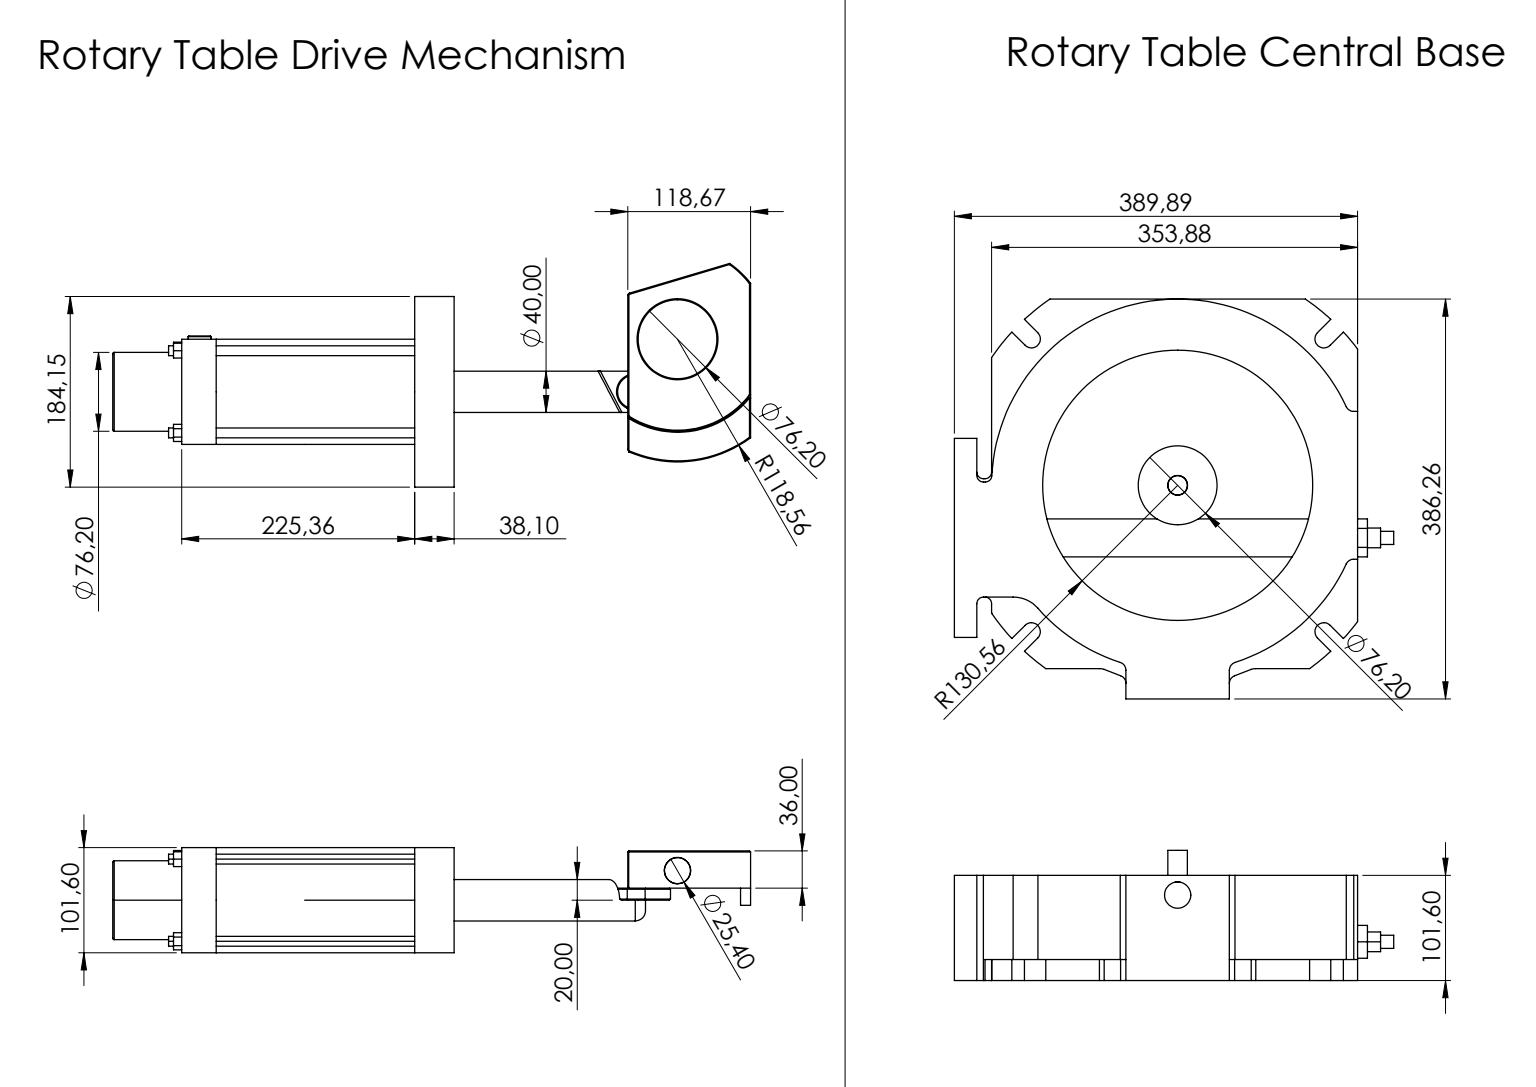
ISO-10303-21;
HEADER;
FILE_DESCRIPTION (('STEP AP214'),
    '1' );
FILE_NAME ('Rotary Table Drive Mechanism.step',
    '2026-10-07T11:37:37',
    ( '' ),
    ( '' ),
    'SwSTEP 2.0',
    'SolidWorks 2020',
    '' );
FILE_SCHEMA (( 'AUTOMOTIVE_DESIGN' ));
ENDSEC;

DATA;
#19=VERTEX_POINT ( 'NONE', #31186 ) ;
#30=CARTESIAN_POINT ( 'NONE',  ( 0.8292115003195463796, 69.84999999999999432, 118.5559999999999832 ) ) ;
#36=DIRECTION ( 'NONE',  ( 0.000000000000000000, 0.000000000000000000, -1.000000000000000000 ) ) ;
#65=DIRECTION ( 'NONE',  ( -0.7071067811865475727, -0.7071067811865475727, 0.000000000000000000 ) ) ;
#72=ADVANCED_FACE ( 'NONE', ( #9419 ), #85748, .F. ) ;
#76=AXIS2_PLACEMENT_3D ( 'NONE', #21854, #16377, #36372 ) ;
#122=DIRECTION ( 'NONE',  ( 0.000000000000000000, -1.000000000000000000, 0.000000000000000000 ) ) ;
#157=DIRECTION ( 'NONE',  ( 1.000000000000000000, 0.000000000000000000, 0.000000000000000000 ) ) ;
#176=DIRECTION ( 'NONE',  ( 1.000000000000000000, 0.000000000000000000, 1.821299053822143307E-16 ) ) ;
#194=AXIS2_PLACEMENT_3D ( 'NONE', #47993, #62984, #27575 ) ;
#207=DIRECTION ( 'NONE',  ( 1.000000000000000000, 0.000000000000000000, 0.000000000000000000 ) ) ;
#214=ORIENTED_EDGE ( 'NONE', *, *, #36681, .T. ) ;
#244=EDGE_CURVE ( 'NONE', #1586, #65784, #48833, .T. ) ;
#274=VERTEX_POINT ( 'NONE', #40238 ) ;
#280=EDGE_CURVE ( 'NONE', #76657, #85611, #63382, .T. ) ;
#296=VERTEX_POINT ( 'NONE', #28870 ) ;
#343=CARTESIAN_POINT ( 'NONE',  ( -479.3614999999999782, 100.8062500000000057, 94.61194598552329182 ) ) ;
#351=LINE ( 'NONE', #55290, #78955 ) ;
#356=DIRECTION ( 'NONE',  ( 0.000000000000000000, 0.000000000000000000, 1.000000000000000000 ) ) ;
#360=DIRECTION ( 'NONE',  ( 0.000000000000000000, 0.000000000000000000, -1.000000000000000000 ) ) ;
#382=EDGE_LOOP ( 'NONE', ( #48463, #62234, #46660, #29247, #79434, #62043 ) ) ;
#393=CARTESIAN_POINT ( 'NONE',  ( -487.2989999999999782, 14.28749999999982201, 90.48749999999999716 ) ) ;
#415=DIRECTION ( 'NONE',  ( 1.000000000000000000, 0.000000000000000000, 0.000000000000000000 ) ) ;
#426=ORIENTED_EDGE ( 'NONE', *, *, #55411, .F. ) ;
#473=CARTESIAN_POINT ( 'NONE',  ( 10.08011576702975809, 74.81331742494347736, 118.1269967869636019 ) ) ;
#480=VECTOR ( 'NONE', #16393, 1000.000000000000000 ) ;
#511=EDGE_LOOP ( 'NONE', ( #26969, #6552, #8684, #42903 ) ) ;
#531=EDGE_LOOP ( 'NONE', ( #19739, #23308, #31403, #15444, #2300 ) ) ;
#545=CARTESIAN_POINT ( 'NONE',  ( 0.4111459596590908983, 95.14999999999999147, 118.3559999999999945 ) ) ;
#552=CARTESIAN_POINT ( 'NONE',  ( 11.93654059743609963, 78.49423263675578255, 117.7526061616926398 ) ) ;
#562=PLANE ( 'NONE',  #46520 ) ;
#566=EDGE_LOOP ( 'NONE', ( #67679, #88603, #1718, #53923 ) ) ;
#571=VECTOR ( 'NONE', #71127, 1000.000000000000000 ) ;
#598=VECTOR ( 'NONE', #63493, 1000.000000000000114 ) ;
#609=FACE_OUTER_BOUND ( 'NONE', #72490, .T. ) ;
#629=CARTESIAN_POINT ( 'NONE',  ( -462.0260000000000105, 53.97500000000000142, -3.174999999999999822 ) ) ;
#632=DIRECTION ( 'NONE',  ( 0.000000000000000000, -1.000000000000000000, 0.000000000000000000 ) ) ;
#665=AXIS2_PLACEMENT_3D ( 'NONE', #8895, #11561, #17475 ) ;
#676=EDGE_CURVE ( 'NONE', #8470, #22374, #75390, .T. ) ;
#683=ORIENTED_EDGE ( 'NONE', *, *, #39535, .T. ) ;
#688=ADVANCED_FACE ( 'NONE', ( #31376, #44999, #10057 ), #30499, .F. ) ;
#702=DIRECTION ( 'NONE',  ( 0.000000000000000000, -1.000000000000000000, 2.048885995248199879E-16 ) ) ;
#737=AXIS2_PLACEMENT_3D ( 'NONE', #66551, #4341, #52876 ) ;
#756=ORIENTED_EDGE ( 'NONE', *, *, #83309, .F. ) ;
#768=CARTESIAN_POINT ( 'NONE',  ( -41.60202597009397607, 76.06518036156089124, 54.55338361873603503 ) ) ;
#771=EDGE_CURVE ( 'NONE', #74494, #28457, #8136, .T. ) ;
#787=ADVANCED_FACE ( 'NONE', ( #7793 ), #6449, .F. ) ;
#813=EDGE_CURVE ( 'NONE', #65108, #77202, #82778, .T. ) ;
#877=VERTEX_POINT ( 'NONE', #75499 ) ;
#900=LINE ( 'NONE', #84028, #66537 ) ;
#908=ORIENTED_EDGE ( 'NONE', *, *, #55610, .T. ) ;
#911=ORIENTED_EDGE ( 'NONE', *, *, #31846, .F. ) ;
#913=ORIENTED_EDGE ( 'NONE', *, *, #78891, .T. ) ;
#925=EDGE_CURVE ( 'NONE', #41798, #56710, #4893, .T. ) ;
#931=AXIS2_PLACEMENT_3D ( 'NONE', #34340, #61592, #6645 ) ;
#938=DIRECTION ( 'NONE',  ( 0.000000000000000000, 1.365923996832131856E-16, -1.000000000000000000 ) ) ;
#970=VERTEX_POINT ( 'NONE', #3995 ) ;
#983=EDGE_CURVE ( 'NONE', #35866, #2341, #17632, .T. ) ;
#1004=VERTEX_POINT ( 'NONE', #15963 ) ;
#1020=ORIENTED_EDGE ( 'NONE', *, *, #22420, .F. ) ;
#1023=DIRECTION ( 'NONE',  ( 0.000000000000000000, 0.000000000000000000, 1.000000000000000000 ) ) ;
#1045=VECTOR ( 'NONE', #50807, 1000.000000000000000 ) ;
#1062=DIRECTION ( 'NONE',  ( 0.000000000000000000, 0.000000000000000000, -1.000000000000000000 ) ) ;
#1096=CARTESIAN_POINT ( 'NONE',  ( -254.0000000000000000, 93.66249999999999432, 15.87500000000039968 ) ) ;
#1116=ORIENTED_EDGE ( 'NONE', *, *, #64438, .T. ) ;
#1131=AXIS2_PLACEMENT_3D ( 'NONE', #86583, #87473, #80666 ) ;
#1164=CARTESIAN_POINT ( 'NONE',  ( -254.0000000000000000, 3.174999999999999822, -41.27499999999999858 ) ) ;
#1175=FACE_OUTER_BOUND ( 'NONE', #74451, .T. ) ;
#1180=DIRECTION ( 'NONE',  ( 0.000000000000000000, 0.000000000000000000, -1.000000000000000000 ) ) ;
#1198=DIRECTION ( 'NONE',  ( 0.000000000000000000, 1.000000000000000000, 0.000000000000000000 ) ) ;
#1199=AXIS2_PLACEMENT_3D ( 'NONE', #57374, #64210, #15161 ) ;
#1204=VECTOR ( 'NONE', #3252, 1000.000000000000114 ) ;
#1209=EDGE_CURVE ( 'NONE', #36892, #42299, #54799, .T. ) ;
#1211=DIRECTION ( 'NONE',  ( 1.000000000000000000, 0.000000000000000000, 0.000000000000000000 ) ) ;
#1223=PLANE ( 'NONE',  #63688 ) ;
#1236=CARTESIAN_POINT ( 'NONE',  ( -53.64297985755450782, 53.97500000000000142, 70.79999999999999716 ) ) ;
#1242=ORIENTED_EDGE ( 'NONE', *, *, #88066, .T. ) ;
#1248=CARTESIAN_POINT ( 'NONE',  ( 0.000000000000000000, 65.60000000000000853, 0.000000000000000000 ) ) ;
#1256=AXIS2_PLACEMENT_3D ( 'NONE', #56524, #84270, #2479 ) ;
#1268=ORIENTED_EDGE ( 'NONE', *, *, #83334, .T. ) ;
#1301=VERTEX_POINT ( 'NONE', #33039 ) ;
#1311=CIRCLE ( 'NONE', #81076, 3.700000000000001954 ) ;
#1312=DIRECTION ( 'NONE',  ( 0.000000000000000000, 0.000000000000000000, -1.000000000000000000 ) ) ;
#1314=DIRECTION ( 'NONE',  ( 0.000000000000000000, -0.7071067811865474617, -0.7071067811865474617 ) ) ;
#1357=LINE ( 'NONE', #85388, #71182 ) ;
#1403=EDGE_CURVE ( 'NONE', #64560, #10945, #72925, .T. ) ;
#1412=ORIENTED_EDGE ( 'NONE', *, *, #75155, .T. ) ;
#1454=CARTESIAN_POINT ( 'NONE',  ( -446.0240000000000009, 14.28749999999982201, 85.72499999999999432 ) ) ;
#1457=DIRECTION ( 'NONE',  ( 0.000000000000000000, 0.000000000000000000, 1.000000000000000000 ) ) ;
#1459=FACE_OUTER_BOUND ( 'NONE', #4609, .T. ) ;
#1462=CARTESIAN_POINT ( 'NONE',  ( -1.790903581468949841E-22, 95.14999999999999147, 118.3560000000000088 ) ) ;
#1472=VERTEX_POINT ( 'NONE', #66554 ) ;
#1477=VECTOR ( 'NONE', #62930, 1000.000000000000000 ) ;
#1487=ORIENTED_EDGE ( 'NONE', *, *, #80879, .F. ) ;
#1516=DIRECTION ( 'NONE',  ( 0.000000000000000000, 0.000000000000000000, 1.000000000000000000 ) ) ;
#1518=LINE ( 'NONE', #42816, #49126 ) ;
#1520=PLANE ( 'NONE',  #1780 ) ;
#1544=CARTESIAN_POINT ( 'NONE',  ( -479.3614999999999782, 97.78694598552380057, 3.968750000000479616 ) ) ;
#1571=VERTEX_POINT ( 'NONE', #18861 ) ;
#1577=CARTESIAN_POINT ( 'NONE',  ( -473.2019999999999982, 53.97500000000000142, -3.174999999999999822 ) ) ;
#1586=VERTEX_POINT ( 'NONE', #81563 ) ;
#1601=DIRECTION ( 'NONE',  ( 1.000000000000000000, 0.000000000000000000, -0.000000000000000000 ) ) ;
#1604=EDGE_CURVE ( 'NONE', #27384, #82662, #81115, .T. ) ;
#1633=CARTESIAN_POINT ( 'NONE',  ( -454.6936515812919879, 53.97500000000000142, -3.174999999999999822 ) ) ;
#1709=ADVANCED_FACE ( 'NONE', ( #34722 ), #56947, .F. ) ;
#1713=CARTESIAN_POINT ( 'NONE',  ( -37.97768777873315571, 53.97499999999997300, 70.36347694520327423 ) ) ;
#1718=ORIENTED_EDGE ( 'NONE', *, *, #34498, .F. ) ;
#1729=CARTESIAN_POINT ( 'NONE',  ( -546.0365000000000464, 53.97500000000000142, 14.22400000000000020 ) ) ;
#1780=AXIS2_PLACEMENT_3D ( 'NONE', #14699, #63285, #70099 ) ;
#1781=DIRECTION ( 'NONE',  ( -1.000000000000000000, 0.000000000000000000, 0.000000000000000000 ) ) ;
#1785=B_SPLINE_CURVE_WITH_KNOTS ( 'NONE', 3,
 ( #11511, #25577, #26926, #53253, #18768, #82360, #20122, #74184, #53704, #60994, #81470, #40095, #47796, #26478, #40993, #68714, #87369, #81910, #25130, #62779, #77774, #14654, #7382, #50036, #56406 ),
 .UNSPECIFIED., .F., .F.,
 ( 4, 2, 2, 2, 2, 2, 2, 2, 2, 1, 2, 2, 4 ),
 ( 0.000000000000000000, 0.002464400387950989747, 0.003696600581926483536, 0.004928800775901976891, 0.007393201163853002633, 0.008625401357828533719, 0.009857601551804066539, 0.01232200193975515994, 0.01355420213373072051, 0.01478640232770627762, 0.01601860252168183646, 0.01725080271565739357, 0.01971520310360850431 ),
 .UNSPECIFIED. ) ;
#1787=ORIENTED_EDGE ( 'NONE', *, *, #17427, .F. ) ;
#1822=DIRECTION ( 'NONE',  ( -0.000000000000000000, 1.000000000000000000, -0.000000000000000000 ) ) ;
#1829=DIRECTION ( 'NONE',  ( 0.000000000000000000, 0.8660254037844383745, -0.5000000000000003331 ) ) ;
#1831=CARTESIAN_POINT ( 'NONE',  ( 11.02121562796429899, 76.18511308578193564, 118.0435185069309227 ) ) ;
#1834=ORIENTED_EDGE ( 'NONE', *, *, #34415, .T. ) ;
#1848=ADVANCED_FACE ( 'NONE', ( #30598 ), #44655, .F. ) ;
#1854=DIRECTION ( 'NONE',  ( 0.5477458065102255302, 0.7071067811865671127, 0.4471851198893302959 ) ) ;
#1863=CARTESIAN_POINT ( 'NONE',  ( -11.65426927613973085, 77.70835675146533106, 117.7811321253428787 ) ) ;
#1867=CARTESIAN_POINT ( 'NONE',  ( -454.6936515812919879, 53.97500000000000142, 3.174999999999999822 ) ) ;
#1883=LINE ( 'NONE', #28686, #81939 ) ;
#1902=CARTESIAN_POINT ( 'NONE',  ( 11.95695845665503043, 86.60868480869159214, 117.7509010089503363 ) ) ;
#1905=ORIENTED_EDGE ( 'NONE', *, *, #30326, .F. ) ;
#1914=CARTESIAN_POINT ( 'NONE',  ( 11.65927451492354550, 77.72029911766621524, 117.7806352395324723 ) ) ;
#1931=CYLINDRICAL_SURFACE ( 'NONE', #10276, 17.33514202138210081 ) ;
#1948=CARTESIAN_POINT ( 'NONE',  ( -487.2989999999999782, 93.66249999999999432, 82.23860802895320887 ) ) ;
#1949=EDGE_CURVE ( 'NONE', #63134, #36007, #78323, .T. ) ;
#1952=VECTOR ( 'NONE', #71675, 1000.000000000000000 ) ;
#1959=AXIS2_PLACEMENT_3D ( 'NONE', #75785, #19470, #26721 ) ;
#1965=CARTESIAN_POINT ( 'NONE',  ( -462.0260000000000105, 53.97500000000000142, -3.174999999999999822 ) ) ;
#1971=VERTEX_POINT ( 'NONE', #79659 ) ;
#1986=LINE ( 'NONE', #16070, #88215 ) ;
#2006=ADVANCED_FACE ( 'NONE', ( #31472, #59176 ), #86906, .F. ) ;
#2024=EDGE_CURVE ( 'NONE', #71038, #26842, #11493, .T. ) ;
#2027=EDGE_LOOP ( 'NONE', ( #79805, #9909, #35090, #9036, #6972, #60590 ) ) ;
#2076=DIRECTION ( 'NONE',  ( 1.000000000000000000, 0.000000000000000000, 0.000000000000000000 ) ) ;
#2077=FACE_OUTER_BOUND ( 'NONE', #12884, .T. ) ;
#2095=CIRCLE ( 'NONE', #4929, 4.762500000000000178 ) ;
#2096=ORIENTED_EDGE ( 'NONE', *, *, #26575, .F. ) ;
#2123=AXIS2_PLACEMENT_3D ( 'NONE', #56026, #28332, #8820 ) ;
#2136=ORIENTED_EDGE ( 'NONE', *, *, #46594, .F. ) ;
#2141=EDGE_CURVE ( 'NONE', #16953, #80801, #53232, .T. ) ;
#2153=ORIENTED_EDGE ( 'NONE', *, *, #73110, .T. ) ;
#2162=VERTEX_POINT ( 'NONE', #60515 ) ;
#2165=EDGE_CURVE ( 'NONE', #24211, #76657, #46873, .T. ) ;
#2181=CARTESIAN_POINT ( 'NONE',  ( -446.0240000000000009, 104.7749999999999915, 50.79999999999999716 ) ) ;
#2226=ORIENTED_EDGE ( 'NONE', *, *, #83708, .F. ) ;
#2230=ORIENTED_EDGE ( 'NONE', *, *, #88066, .F. ) ;
#2259=ORIENTED_EDGE ( 'NONE', *, *, #67555, .F. ) ;
#2262=ORIENTED_EDGE ( 'NONE', *, *, #58636, .F. ) ;
#2269=CARTESIAN_POINT ( 'NONE',  ( -462.0260000000000105, 53.97500000000000142, -2.412999999999919876 ) ) ;
#2276=CARTESIAN_POINT ( 'NONE',  ( -48.67264380398864176, 64.60000000000000853, 66.68100227564391957 ) ) ;
#2300=ORIENTED_EDGE ( 'NONE', *, *, #74106, .T. ) ;
#2325=EDGE_LOOP ( 'NONE', ( #59045, #35444 ) ) ;
#2341=VERTEX_POINT ( 'NONE', #1454 ) ;
#2346=CARTESIAN_POINT ( 'NONE',  ( -473.2019999999999982, 53.97500000000000142, -1.387778780781445991E-14 ) ) ;
#2397=FACE_OUTER_BOUND ( 'NONE', #40658, .T. ) ;
#2403=EDGE_CURVE ( 'NONE', #22043, #36708, #81778, .T. ) ;
#2412=CARTESIAN_POINT ( 'NONE',  ( -469.3583484187089994, 53.97500000000000142, -3.174999999999999822 ) ) ;
#2415=DIRECTION ( 'NONE',  ( 1.000000000000000000, 0.000000000000000000, 0.000000000000000000 ) ) ;
#2479=DIRECTION ( 'NONE',  ( 0.000000000000000000, 0.000000000000000000, -1.000000000000000000 ) ) ;
#2568=DIRECTION ( 'NONE',  ( 0.000000000000000000, 0.000000000000000000, 1.000000000000000000 ) ) ;
#2569=DIRECTION ( 'NONE',  ( -1.000000000000000000, 0.000000000000000000, 0.000000000000000000 ) ) ;
#2600=EDGE_LOOP ( 'NONE', ( #46917, #45524, #28204, #67495 ) ) ;
#2613=ORIENTED_EDGE ( 'NONE', *, *, #68493, .T. ) ;
#2656=AXIS2_PLACEMENT_3D ( 'NONE', #36792, #63601, #44476 ) ;
#2678=ORIENTED_EDGE ( 'NONE', *, *, #5270, .T. ) ;
#2687=ORIENTED_EDGE ( 'NONE', *, *, #76279, .T. ) ;
#2704=DIRECTION ( 'NONE',  ( 0.000000000000000000, -0.000000000000000000, 1.000000000000000000 ) ) ;
#2769=DIRECTION ( 'NONE',  ( -1.000000000000000000, 0.000000000000000000, 0.000000000000000000 ) ) ;
#2792=DIRECTION ( 'NONE',  ( 1.000000000000000000, 0.000000000000000000, 0.000000000000000000 ) ) ;
#2796=FACE_OUTER_BOUND ( 'NONE', #75278, .T. ) ;
#2799=LINE ( 'NONE', #44102, #58933 ) ;
#2801=CARTESIAN_POINT ( 'NONE',  ( 12.57992033961893341, 83.37360573934186903, 117.6855557170023019 ) ) ;
#2843=EDGE_LOOP ( 'NONE', ( #38287, #47019, #30923, #33243 ) ) ;
#2860=EDGE_CURVE ( 'NONE', #50592, #42067, #14600, .T. ) ;
#2892=ORIENTED_EDGE ( 'NONE', *, *, #72960, .T. ) ;
#2903=CARTESIAN_POINT ( 'NONE',  ( -12.70000000000000107, 82.54999999999999716, 117.8738102209307641 ) ) ;
#2918=CARTESIAN_POINT ( 'NONE',  ( -30.89999999999999858, 53.97500000000000142, 50.79999999999999716 ) ) ;
#2949=VERTEX_POINT ( 'NONE', #79226 ) ;
#2958=CARTESIAN_POINT ( 'NONE',  ( -487.2989999999999782, 21.43125000000035030, 6.988054014476359654 ) ) ;
#3017=EDGE_CURVE ( 'NONE', #32697, #73034, #89030, .T. ) ;
#3020=CARTESIAN_POINT ( 'NONE',  ( -446.0240000000000009, 93.66249999999999432, 90.48749999999999716 ) ) ;
#3031=CARTESIAN_POINT ( 'NONE',  ( -487.2989999999999782, 22.53639197104660141, 90.48749999999999716 ) ) ;
#3052=PLANE ( 'NONE',  #49461 ) ;
#3058=DIRECTION ( 'NONE',  ( 0.000000000000000000, -0.000000000000000000, 1.000000000000000000 ) ) ;
#3061=DIRECTION ( 'NONE',  ( 0.3182345505295408605, 0.3182345505294081889, -0.8930025429407280058 ) ) ;
#3063=CARTESIAN_POINT ( 'NONE',  ( -479.3614999999999782, 53.97500000000000142, 50.79999999999999716 ) ) ;
#3100=CARTESIAN_POINT ( 'NONE',  ( -492.0614999999999668, 14.28750000000026077, 15.87499999999969802 ) ) ;
#3146=EDGE_CURVE ( 'NONE', #19524, #58138, #56850, .T. ) ;
#3157=DIRECTION ( 'NONE',  ( 0.000000000000000000, 0.4999999999999995004, 0.8660254037844390407 ) ) ;
#3167=DIRECTION ( 'NONE',  ( -0.9770521142508956647, -0.000000000000000000, 0.2130003897598659046 ) ) ;
#3169=EDGE_CURVE ( 'NONE', #75163, #32749, #49582, .T. ) ;
#3175=FACE_OUTER_BOUND ( 'NONE', #62080, .T. ) ;
#3207=VECTOR ( 'NONE', #82179, 1000.000000000000000 ) ;
#3230=ORIENTED_EDGE ( 'NONE', *, *, #31735, .F. ) ;
#3244=CARTESIAN_POINT ( 'NONE',  ( -31.27367473141074683, 148.4450814996825443, 74.45358409497265484 ) ) ;
#3247=CARTESIAN_POINT ( 'NONE',  ( 10.08805235722132565, 90.30997682696688855, 118.1269383658995338 ) ) ;
#3252=DIRECTION ( 'NONE',  ( 0.9130365726098600421, 0.000000000000000000, 0.4078776986755215939 ) ) ;
#3253=CARTESIAN_POINT ( 'NONE',  ( -465.6921742093550165, 47.62500000000000000, 3.174999999999999822 ) ) ;
#3273=PLANE ( 'NONE',  #49425 ) ;
#3303=FACE_OUTER_BOUND ( 'NONE', #82744, .T. ) ;
#3313=FACE_OUTER_BOUND ( 'NONE', #54090, .T. ) ;
#3353=VERTEX_POINT ( 'NONE', #3253 ) ;
#3401=LINE ( 'NONE', #46493, #50803 ) ;
#3404=CARTESIAN_POINT ( 'NONE',  ( 70.63919639214310564, 65.60000000000000853, 95.21359708083839735 ) ) ;
#3429=ORIENTED_EDGE ( 'NONE', *, *, #25778, .T. ) ;
#3433=ORIENTED_EDGE ( 'NONE', *, *, #35404, .F. ) ;
#3447=CARTESIAN_POINT ( 'NONE',  ( -446.0240000000000009, 53.97500000000000142, -1.387778780781445991E-14 ) ) ;
#3450=EDGE_CURVE ( 'NONE', #51171, #80177, #61760, .T. ) ;
#3487=EDGE_LOOP ( 'NONE', ( #22652, #78379, #77739, #75778 ) ) ;
#3495=CARTESIAN_POINT ( 'NONE',  ( 70.63919639214310564, 100.5999999999999659, 56.85413200336923012 ) ) ;
#3498=VECTOR ( 'NONE', #48714, 1000.000000000000114 ) ;
#3529=VECTOR ( 'NONE', #59244, 1000.000000000000114 ) ;
#3558=CIRCLE ( 'NONE', #22446, 4.762500000000000178 ) ;
#3587=AXIS2_PLACEMENT_3D ( 'NONE', #87118, #79875, #44874 ) ;
#3588=AXIS2_PLACEMENT_3D ( 'NONE', #82069, #47499, #84753 ) ;
#3639=EDGE_CURVE ( 'NONE', #77842, #64816, #77212, .T. ) ;
#3682=CARTESIAN_POINT ( 'NONE',  ( 11.39249797916225759, 88.17791239546554038, 118.0075204203976114 ) ) ;
#3683=EDGE_LOOP ( 'NONE', ( #37779, #86747, #48970, #84441 ) ) ;
#3701=LINE ( 'NONE', #74532, #55266 ) ;
#3722=DIRECTION ( 'NONE',  ( 0.000000000000000000, 0.000000000000000000, -1.000000000000000000 ) ) ;
#3737=VECTOR ( 'NONE', #84099, 1000.000000000000000 ) ;
#3742=EDGE_CURVE ( 'NONE', #75550, #1586, #63574, .T. ) ;
#3788=CARTESIAN_POINT ( 'NONE',  ( -12.29201543513789652, 79.25066774386124280, 117.9171666014395043 ) ) ;
#3793=ORIENTED_EDGE ( 'NONE', *, *, #73379, .T. ) ;
#3812=CARTESIAN_POINT ( 'NONE',  ( -446.0240000000000009, 53.97500000000000142, 101.5999999999999943 ) ) ;
#3820=DIRECTION ( 'NONE',  ( 0.000000000000000000, -1.000000000000000000, 0.000000000000000000 ) ) ;
#3853=ADVANCED_FACE ( 'NONE', ( #45336 ), #44451, .T. ) ;
#3877=ORIENTED_EDGE ( 'NONE', *, *, #33688, .F. ) ;
#3913=EDGE_LOOP ( 'NONE', ( #31915, #88377, #7942 ) ) ;
#3922=AXIS2_PLACEMENT_3D ( 'NONE', #47491, #67058, #74771 ) ;
#3935=CARTESIAN_POINT ( 'NONE',  ( 1.796236281188243881E-22, 69.84999999999999432, 118.5560000000000116 ) ) ;
#3942=CARTESIAN_POINT ( 'NONE',  ( -446.0240000000000009, 3.174999999999999822, -1.387778780781445991E-14 ) ) ;
#3995=CARTESIAN_POINT ( 'NONE',  ( -487.2989999999999782, 18.41194598552324990, 83.34375000000000000 ) ) ;
#4010=CARTESIAN_POINT ( 'NONE',  ( -8.690350657389011246, 91.82034414994009808, 118.2374269007433440 ) ) ;
#4021=DIRECTION ( 'NONE',  ( 0.9130365726098600421, -0.000000000000000000, 0.4078776986755216494 ) ) ;
#4027=CARTESIAN_POINT ( 'NONE',  ( -48.67264380398864176, 54.97499999999996589, 66.68100227564391957 ) ) ;
#4045=EDGE_CURVE ( 'NONE', #78144, #37970, #73960, .T. ) ;
#4068=EDGE_CURVE ( 'NONE', #54103, #41996, #66232, .T. ) ;
#4086=EDGE_CURVE ( 'NONE', #81729, #45431, #45779, .T. ) ;
#4097=DIRECTION ( 'NONE',  ( 0.9130365726098600421, 0.000000000000000000, 0.4078776986755215939 ) ) ;
#4123=ORIENTED_EDGE ( 'NONE', *, *, #34464, .T. ) ;
#4134=CARTESIAN_POINT ( 'NONE',  ( 4.052643387441906775, 70.61235367433147303, 118.2872599129365057 ) ) ;
#4140=ORIENTED_EDGE ( 'NONE', *, *, #28041, .T. ) ;
#4155=ORIENTED_EDGE ( 'NONE', *, *, #70123, .T. ) ;
#4157=ADVANCED_FACE ( 'NONE', ( #68042, #19892 ), #42550, .T. ) ;
#4191=VECTOR ( 'NONE', #3167, 1000.000000000000114 ) ;
#4194=EDGE_CURVE ( 'NONE', #8698, #37391, #44436, .T. ) ;
#4231=AXIS2_PLACEMENT_3D ( 'NONE', #29075, #15456, #57206 ) ;
#4232=CARTESIAN_POINT ( 'NONE',  ( -4.091298994373309128, 70.49827730944788584, 118.4878841633551474 ) ) ;
#4275=AXIS2_PLACEMENT_3D ( 'NONE', #27906, #57398, #8832 ) ;
#4280=DIRECTION ( 'NONE',  ( 0.000000000000000000, 0.000000000000000000, 1.000000000000000000 ) ) ;
#4282=EDGE_CURVE ( 'NONE', #36892, #34120, #15326, .T. ) ;
#4287=AXIS2_PLACEMENT_3D ( 'NONE', #39761, #68388, #20237 ) ;
#4294=DIRECTION ( 'NONE',  ( 0.000000000000000000, 0.000000000000000000, 1.000000000000000000 ) ) ;
#4303=LINE ( 'NONE', #38361, #41347 ) ;
#4328=ORIENTED_EDGE ( 'NONE', *, *, #59587, .F. ) ;
#4337=VECTOR ( 'NONE', #55934, 1000.000000000000000 ) ;
#4341=DIRECTION ( 'NONE',  ( -1.000000000000000000, 0.000000000000000000, 0.000000000000000000 ) ) ;
#4366=ADVANCED_FACE ( 'NONE', ( #65254 ), #23928, .F. ) ;
#4367=ORIENTED_EDGE ( 'NONE', *, *, #33334, .F. ) ;
#4399=DIRECTION ( 'NONE',  ( 0.000000000000000000, 1.000000000000000000, 0.000000000000000000 ) ) ;
#4427=FACE_OUTER_BOUND ( 'NONE', #35154, .T. ) ;
#4464=CARTESIAN_POINT ( 'NONE',  ( -5.634993000313458289, 93.96183429002098819, 118.4245090560989837 ) ) ;
#4483=ORIENTED_EDGE ( 'NONE', *, *, #77723, .F. ) ;
#4518=DIRECTION ( 'NONE',  ( -0.000000000000000000, -1.000000000000000000, -0.000000000000000000 ) ) ;
#4522=ORIENTED_EDGE ( 'NONE', *, *, #26681, .T. ) ;
#4574=FACE_OUTER_BOUND ( 'NONE', #30067, .T. ) ;
#4590=VECTOR ( 'NONE', #84397, 1000.000000000000000 ) ;
#4604=CARTESIAN_POINT ( 'NONE',  ( -487.2989999999999782, 100.8062500000000057, 86.36305401447658880 ) ) ;
#4609=EDGE_LOOP ( 'NONE', ( #82337, #46693, #74543, #83845 ) ) ;
#4620=ORIENTED_EDGE ( 'NONE', *, *, #46310, .T. ) ;
#4633=CARTESIAN_POINT ( 'NONE',  ( -487.2989999999999782, 97.78694598552370110, 18.25625000000050235 ) ) ;
#4645=CIRCLE ( 'NONE', #55385, 4.762500000000000178 ) ;
#4649=VECTOR ( 'NONE', #45141, 1000.000000000000000 ) ;
#4685=DIRECTION ( 'NONE',  ( 0.000000000000000000, 0.000000000000000000, 1.000000000000000000 ) ) ;
#4705=CARTESIAN_POINT ( 'NONE',  ( -15.88716625750469902, 91.07499999999996021, -53.54073290201169044 ) ) ;
#4706=ADVANCED_FACE ( 'NONE', ( #33709 ), #32345, .T. ) ;
#4733=AXIS2_PLACEMENT_3D ( 'NONE', #50180, #43366, #16579 ) ;
#4746=VECTOR ( 'NONE', #74236, 1000.000000000000000 ) ;
#4759=DIRECTION ( 'NONE',  ( 0.000000000000000000, 0.000000000000000000, -1.000000000000000000 ) ) ;
#4762=CARTESIAN_POINT ( 'NONE',  ( 69.63919639214307722, 92.07499999999998863, 53.63573739454427880 ) ) ;
#4807=VERTEX_POINT ( 'NONE', #11544 ) ;
#4863=CARTESIAN_POINT ( 'NONE',  ( 70.63919639214310564, 91.07499999999996021, 53.63573739454427880 ) ) ;
#4893=LINE ( 'NONE', #79877, #11248 ) ;
#4929=AXIS2_PLACEMENT_3D ( 'NONE', #46373, #67741, #39575 ) ;
#4932=CARTESIAN_POINT ( 'NONE',  ( -492.0614999999999668, 14.28749999999982201, 90.48749999999999716 ) ) ;
#4958=ORIENTED_EDGE ( 'NONE', *, *, #85234, .F. ) ;
#4961=DIRECTION ( 'NONE',  ( 0.000000000000000000, 0.000000000000000000, -1.000000000000000000 ) ) ;
#4988=DIRECTION ( 'NONE',  ( 0.000000000000000000, 0.000000000000000000, -1.000000000000000000 ) ) ;
#5001=LINE ( 'NONE', #12264, #5018 ) ;
#5008=VECTOR ( 'NONE', #32730, 1000.000000000000114 ) ;
#5018=VECTOR ( 'NONE', #39958, 1000.000000000000000 ) ;
#5029=CARTESIAN_POINT ( 'NONE',  ( -492.0614999999999668, 93.66249999999999432, 90.48749999999999716 ) ) ;
#5032=LINE ( 'NONE', #11851, #84848 ) ;
#5148=CARTESIAN_POINT ( 'NONE',  ( -254.0000000000000000, 93.66249999999999432, 95.25000000000000000 ) ) ;
#5213=ORIENTED_EDGE ( 'NONE', *, *, #41344, .F. ) ;
#5260=LINE ( 'NONE', #5719, #32735 ) ;
#5270=EDGE_CURVE ( 'NONE', #88352, #83829, #83961, .T. ) ;
#5280=LINE ( 'NONE', #25262, #55233 ) ;
#5289=ORIENTED_EDGE ( 'NONE', *, *, #45576, .T. ) ;
#5292=DIRECTION ( 'NONE',  ( 0.000000000000000000, -0.8660254037844432595, 0.4999999999999921174 ) ) ;
#5301=CARTESIAN_POINT ( 'NONE',  ( -492.0614999999999668, 14.28749999999982201, 90.48749999999999716 ) ) ;
#5322=CARTESIAN_POINT ( 'NONE',  ( -50.35902679310718355, 148.4450814996825443, 27.95514712793348977 ) ) ;
#5359=CARTESIAN_POINT ( 'NONE',  ( -10.09401914261505517, 90.30230937457700691, 118.1264283250772564 ) ) ;
#5362=CARTESIAN_POINT ( 'NONE',  ( -47.02966122971771767, 65.60000000000000853, -44.00307561052233751 ) ) ;
#5391=DIRECTION ( 'NONE',  ( -1.000000000000000000, 0.000000000000000000, 0.000000000000000000 ) ) ;
#5401=PLANE ( 'NONE',  #1959 ) ;
#5404=VECTOR ( 'NONE', #79234, 1000.000000000000000 ) ;
#5446=AXIS2_PLACEMENT_3D ( 'NONE', #1248, #35749, #56176 ) ;
#5453=LINE ( 'NONE', #87671, #40011 ) ;
#5464=VECTOR ( 'NONE', #21761, 1000.000000000000000 ) ;
#5471=CARTESIAN_POINT ( 'NONE',  ( -41.60202597009397607, 65.59999999999998010, 50.85338361873603219 ) ) ;
#5500=LINE ( 'NONE', #53605, #14427 ) ;
#5522=EDGE_CURVE ( 'NONE', #59384, #8859, #64095, .T. ) ;
#5561=ORIENTED_EDGE ( 'NONE', *, *, #72944, .T. ) ;
#5563=DIRECTION ( 'NONE',  ( -0.9130365726098601531, 0.000000000000000000, -0.4078776986755215384 ) ) ;
#5598=ORIENTED_EDGE ( 'NONE', *, *, #3017, .T. ) ;
#5614=ORIENTED_EDGE ( 'NONE', *, *, #64657, .F. ) ;
#5623=ORIENTED_EDGE ( 'NONE', *, *, #79508, .F. ) ;
#5642=DIRECTION ( 'NONE',  ( 1.000000000000000000, 0.000000000000000000, 0.000000000000000000 ) ) ;
#5651=DIRECTION ( 'NONE',  ( 0.000000000000000000, -1.000000000000000000, 0.000000000000000000 ) ) ;
#5652=DIRECTION ( 'NONE',  ( 1.000000000000000000, 0.000000000000000000, 0.000000000000000000 ) ) ;
#5671=ORIENTED_EDGE ( 'NONE', *, *, #63009, .T. ) ;
#5674=LINE ( 'NONE', #88796, #89401 ) ;
#5676=CARTESIAN_POINT ( 'NONE',  ( -254.0000000000000000, 14.28750000000026077, 6.349999999999710099 ) ) ;
#5686=ORIENTED_EDGE ( 'NONE', *, *, #55498, .F. ) ;
#5691=LINE ( 'NONE', #75170, #23008 ) ;
#5706=CIRCLE ( 'NONE', #78272, 36.57600000000000051 ) ;
#5719=CARTESIAN_POINT ( 'NONE',  ( 69.63919639214310564, 101.5999999999999943, 0.000000000000000000 ) ) ;
#5773=DIRECTION ( 'NONE',  ( -0.4078776986755215384, 0.000000000000000000, 0.9130365726098602641 ) ) ;
#5804=PRODUCT_DEFINITION_FORMATION_WITH_SPECIFIED_SOURCE ( 'ANY', '', #11164, .NOT_KNOWN. ) ;
#5836=ORIENTED_EDGE ( 'NONE', *, *, #31797, .T. ) ;
#5843=ADVANCED_FACE ( 'NONE', ( #70213 ), #69768, .T. ) ;
#5855=CIRCLE ( 'NONE', #29008, 38.10000000000000142 ) ;
#5870=CIRCLE ( 'NONE', #29073, 50.79999999999999716 ) ;
#5911=CARTESIAN_POINT ( 'NONE',  ( -487.2989999999999782, 21.43125000000029701, 15.23694598552314972 ) ) ;
#5921=DIRECTION ( 'NONE',  ( 0.000000000000000000, -1.000000000000000000, 0.000000000000000000 ) ) ;
#5950=CIRCLE ( 'NONE', #8878, 4.762500000000000178 ) ;
#5981=CARTESIAN_POINT ( 'NONE',  ( -34.93928583487483763, 65.60000000000000853, 35.93880153443800651 ) ) ;
#5996=CARTESIAN_POINT ( 'NONE',  ( -0.8322931907936803597, 69.95000000000001705, 118.3559999999999519 ) ) ;
#6006=CARTESIAN_POINT ( 'NONE',  ( 0.000000000000000000, 92.07499999999998863, 39.10000000000005116 ) ) ;
#6015=EDGE_LOOP ( 'NONE', ( #61285, #39036, #56974, #71418 ) ) ;
#6071=ORIENTED_EDGE ( 'NONE', *, *, #10614, .T. ) ;
#6101=VECTOR ( 'NONE', #34390, 1000.000000000000000 ) ;
#6114=CARTESIAN_POINT ( 'NONE',  ( -465.6921742093539933, 60.32499999999999574, -3.174999999999999822 ) ) ;
#6121=LINE ( 'NONE', #73807, #22688 ) ;
#6123=LINE ( 'NONE', #53328, #25685 ) ;
#6203=FACE_OUTER_BOUND ( 'NONE', #78703, .T. ) ;
#6215=DIRECTION ( 'NONE',  ( -1.000000000000000000, 0.000000000000000000, 0.000000000000000000 ) ) ;
#6217=DIRECTION ( 'NONE',  ( 0.000000000000000000, 0.000000000000000000, 1.000000000000000000 ) ) ;
#6220=CARTESIAN_POINT ( 'NONE',  ( -487.2989999999999782, 86.51875000000001137, 94.61194598552339130 ) ) ;
#6244=EDGE_CURVE ( 'NONE', #81257, #74753, #51042, .T. ) ;
#6260=EDGE_LOOP ( 'NONE', ( #79761, #49258, #35291, #60478 ) ) ;
#6269=LINE ( 'NONE', #343, #54088 ) ;
#6272=ADVANCED_FACE ( 'NONE', ( #62379, #41476 ), #1520, .T. ) ;
#6288=EDGE_CURVE ( 'NONE', #72100, #74329, #50086, .T. ) ;
#6314=CARTESIAN_POINT ( 'NONE',  ( -458.3598257906459708, 47.62500000000000000, -3.174999999999999822 ) ) ;
#6326=DIRECTION ( 'NONE',  ( -0.000000000000000000, 1.000000000000000000, -0.000000000000000000 ) ) ;
#6331=CIRCLE ( 'NONE', #59991, 4.762500000000001066 ) ;
#6332=ORIENTED_EDGE ( 'NONE', *, *, #9029, .T. ) ;
#6341=ADVANCED_FACE ( 'NONE', ( #3303 ), #45491, .T. ) ;
#6358=ORIENTED_EDGE ( 'NONE', *, *, #42537, .F. ) ;
#6367=FACE_OUTER_BOUND ( 'NONE', #77444, .T. ) ;
#6378=ORIENTED_EDGE ( 'NONE', *, *, #85745, .F. ) ;
#6388=ORIENTED_EDGE ( 'NONE', *, *, #79508, .T. ) ;
#6401=LINE ( 'NONE', #42252, #8454 ) ;
#6427=ORIENTED_EDGE ( 'NONE', *, *, #18510, .F. ) ;
#6434=LINE ( 'NONE', #47751, #46462 ) ;
#6449=CYLINDRICAL_SURFACE ( 'NONE', #33035, 38.10000000000000142 ) ;
#6478=ORIENTED_EDGE ( 'NONE', *, *, #12450, .T. ) ;
#6511=CARTESIAN_POINT ( 'NONE',  ( -458.3598257906459708, 47.62500000000000000, 3.174999999999999822 ) ) ;
#6523=( NAMED_UNIT ( * ) PLANE_ANGLE_UNIT ( ) SI_UNIT ( $, .RADIAN. ) );
#6551=DIRECTION ( 'NONE',  ( 1.000000000000000000, 0.000000000000000000, 0.000000000000000000 ) ) ;
#6552=ORIENTED_EDGE ( 'NONE', *, *, #75938, .F. ) ;
#6559=CARTESIAN_POINT ( 'NONE',  ( -47.05489187827554076, 92.24160055789619150, 74.44168661866966374 ) ) ;
#6600=CARTESIAN_POINT ( 'NONE',  ( -48.02966122971776741, 91.07499999999996021, 74.26049396966043048 ) ) ;
#6622=ORIENTED_EDGE ( 'NONE', *, *, #13910, .T. ) ;
#6645=DIRECTION ( 'NONE',  ( 0.000000000000000000, 0.000000000000000000, 1.000000000000000000 ) ) ;
#6679=EDGE_CURVE ( 'NONE', #53803, #54103, #34118, .T. ) ;
#6683=LINE ( 'NONE', #89825, #34261 ) ;
#6705=CARTESIAN_POINT ( 'NONE',  ( -47.08814856060967458, 100.9334351204065001, 108.4402773162242823 ) ) ;
#6718=VERTEX_POINT ( 'NONE', #14597 ) ;
#6730=DIRECTION ( 'NONE',  ( 0.000000000000000000, 0.000000000000000000, 1.000000000000000000 ) ) ;
#6754=ORIENTED_EDGE ( 'NONE', *, *, #15746, .F. ) ;
#6772=LINE ( 'NONE', #55346, #59560 ) ;
#6804=ORIENTED_EDGE ( 'NONE', *, *, #34638, .T. ) ;
#6823=AXIS2_PLACEMENT_3D ( 'NONE', #77995, #8502, #58417 ) ;
#6837=CARTESIAN_POINT ( 'NONE',  ( 6.349546116388139261, 71.54336850463093356, 118.3864143103247812 ) ) ;
#6868=CARTESIAN_POINT ( 'NONE',  ( 0.000000000000000000, 353.0471713899363522, 0.000000000000000000 ) ) ;
#6881=DIRECTION ( 'NONE',  ( 1.000000000000000000, 0.000000000000000000, 0.000000000000000000 ) ) ;
#6892=CARTESIAN_POINT ( 'NONE',  ( 0.000000000000000000, 65.60000000000000853, 0.000000000000000000 ) ) ;
#6917=ORIENTED_EDGE ( 'NONE', *, *, #58349, .T. ) ;
#6926=EDGE_CURVE ( 'NONE', #17700, #2162, #72691, .T. ) ;
#6941=CYLINDRICAL_SURFACE ( 'NONE', #84131, 4.762500000000002842 ) ;
#6966=ADVANCED_FACE ( 'NONE', ( #54774 ), #34805, .F. ) ;
#6972=ORIENTED_EDGE ( 'NONE', *, *, #47399, .F. ) ;
#6985=LINE ( 'NONE', #28306, #18761 ) ;
#6992=CARTESIAN_POINT ( 'NONE',  ( -45.51636842011945561, 65.60000000000000853, -45.51636842012056405 ) ) ;
#7001=VERTEX_POINT ( 'NONE', #19840 ) ;
#7024=EDGE_CURVE ( 'NONE', #75662, #21236, #20302, .T. ) ;
#7052=ORIENTED_EDGE ( 'NONE', *, *, #50031, .T. ) ;
#7079=VECTOR ( 'NONE', #84196, 1000.000000000000000 ) ;
#7084=DIRECTION ( 'NONE',  ( 1.000000000000000000, 0.000000000000000000, 0.000000000000000000 ) ) ;
#7101=CARTESIAN_POINT ( 'NONE',  ( -48.02966122971777452, 66.60000000000003695, 108.3913132043271617 ) ) ;
#7118=LINE ( 'NONE', #35703, #73125 ) ;
#7129=ORIENTED_EDGE ( 'NONE', *, *, #9959, .F. ) ;
#7146=ORIENTED_EDGE ( 'NONE', *, *, #86511, .T. ) ;
#7158=VERTEX_POINT ( 'NONE', #24754 ) ;
#7176=VECTOR ( 'NONE', #78493, 1000.000000000000000 ) ;
#7189=AXIS2_PLACEMENT_3D ( 'NONE', #25118, #11042, #19646 ) ;
#7195=CARTESIAN_POINT ( 'NONE',  ( 69.47395303589517823, 92.29081221604221241, 54.20185447853388894 ) ) ;
#7210=DIRECTION ( 'NONE',  ( -1.000000000000000000, 0.000000000000000000, 0.000000000000000000 ) ) ;
#7245=ADVANCED_FACE ( 'NONE', ( #79743, #72904 ), #52857, .F. ) ;
#7246=CARTESIAN_POINT ( 'NONE',  ( -254.0000000000000000, 104.7749999999999915, 142.8750000000000000 ) ) ;
#7248=CARTESIAN_POINT ( 'NONE',  ( -76.76533072354217779, 55.69843073979289727, 30.87393032424260753 ) ) ;
#7249=ORIENTED_EDGE ( 'NONE', *, *, #89219, .F. ) ;
#7265=EDGE_LOOP ( 'NONE', ( #54230, #18485, #1020 ) ) ;
#7299=AXIS2_PLACEMENT_3D ( 'NONE', #68980, #21738, #13564 ) ;
#7303=ORIENTED_EDGE ( 'NONE', *, *, #48623, .T. ) ;
#7312=ORIENTED_EDGE ( 'NONE', *, *, #10778, .T. ) ;
#7317=DIRECTION ( 'NONE',  ( 1.821299053822143307E-16, 0.000000000000000000, -1.000000000000000000 ) ) ;
#7359=CARTESIAN_POINT ( 'NONE',  ( -446.0240000000000009, 3.174999999999999822, -1.387778780781445991E-14 ) ) ;
#7378=CIRCLE ( 'NONE', #56637, 4.762500000000002842 ) ;
#7382=CARTESIAN_POINT ( 'NONE',  ( -1.640892575522350905, 95.07020838220610415, 118.3474229726581939 ) ) ;
#7447=ADVANCED_FACE ( 'NONE', ( #81536, #61947 ), #76032, .T. ) ;
#7471=PLANE ( 'NONE',  #9953 ) ;
#7486=DIRECTION ( 'NONE',  ( 0.000000000000000000, 0.000000000000000000, 1.000000000000000000 ) ) ;
#7500=ORIENTED_EDGE ( 'NONE', *, *, #38690, .T. ) ;
#7534=CARTESIAN_POINT ( 'NONE',  ( 68.86456684384336313, 353.0471713899363522, 56.22171674193015178 ) ) ;
#7558=PLANE ( 'NONE',  #9741 ) ;
#7564=ORIENTED_EDGE ( 'NONE', *, *, #39208, .F. ) ;
#7595=ADVANCED_FACE ( 'NONE', ( #63301 ), #16059, .F. ) ;
#7600=CIRCLE ( 'NONE', #68480, 50.79999999999999716 ) ;
#7602=VECTOR ( 'NONE', #28422, 1000.000000000000000 ) ;
#7632=AXIS2_PLACEMENT_3D ( 'NONE', #19110, #14090, #7723 ) ;
#7633=PLANE ( 'NONE',  #56164 ) ;
#7646=VERTEX_POINT ( 'NONE', #64207 ) ;
#7647=CARTESIAN_POINT ( 'NONE',  ( -41.60202597009397607, 54.97499999999995879, 33.51824159735392783 ) ) ;
#7689=DIRECTION ( 'NONE',  ( 0.000000000000000000, 0.6088800793514597132, 0.7932622825831063818 ) ) ;
#7694=PLANE ( 'NONE',  #29253 ) ;
#7702=DIRECTION ( 'NONE',  ( 0.000000000000000000, 0.000000000000000000, -1.000000000000000000 ) ) ;
#7718=AXIS2_PLACEMENT_3D ( 'NONE', #40812, #47167, #20393 ) ;
#7723=DIRECTION ( 'NONE',  ( 0.000000000000000000, 0.000000000000000000, -1.000000000000000000 ) ) ;
#7732=CARTESIAN_POINT ( 'NONE',  ( -41.60202597009397607, 54.97499999999995879, 50.85338361873603219 ) ) ;
#7738=CARTESIAN_POINT ( 'NONE',  ( 11.89015833661310850, 78.06809816022375514, 117.9583611672943277 ) ) ;
#7775=EDGE_LOOP ( 'NONE', ( #22072, #31962, #50120, #49364 ) ) ;
#7790=ORIENTED_EDGE ( 'NONE', *, *, #88880, .F. ) ;
#7792=FACE_OUTER_BOUND ( 'NONE', #47351, .T. ) ;
#7793=FACE_OUTER_BOUND ( 'NONE', #57939, .T. ) ;
#7803=CARTESIAN_POINT ( 'NONE',  ( -479.3614999999999782, 14.28750000000023945, 19.36139197104649767 ) ) ;
#7824=EDGE_CURVE ( 'NONE', #56124, #22947, #87768, .T. ) ;
#7837=ORIENTED_EDGE ( 'NONE', *, *, #15525, .T. ) ;
#7852=EDGE_CURVE ( 'NONE', #2949, #67327, #5950, .T. ) ;
#7854=DIRECTION ( 'NONE',  ( 0.000000000000000000, 0.000000000000000000, -1.000000000000000000 ) ) ;
#7870=DIRECTION ( 'NONE',  ( 0.000000000000000000, 0.000000000000000000, 1.000000000000000000 ) ) ;
#7877=DIRECTION ( 'NONE',  ( -1.000000000000000000, 0.000000000000000000, 0.000000000000000000 ) ) ;
#7896=ORIENTED_EDGE ( 'NONE', *, *, #89251, .F. ) ;
#7908=VERTEX_POINT ( 'NONE', #11466 ) ;
#7922=ORIENTED_EDGE ( 'NONE', *, *, #1403, .F. ) ;
#7926=DIRECTION ( 'NONE',  ( 0.000000000000000000, 0.000000000000000000, -1.000000000000000000 ) ) ;
#7942=ORIENTED_EDGE ( 'NONE', *, *, #45195, .F. ) ;
#7956=EDGE_CURVE ( 'NONE', #38989, #12332, #74142, .T. ) ;
#7988=EDGE_CURVE ( 'NONE', #30366, #80402, #56811, .T. ) ;
#8054=EDGE_CURVE ( 'NONE', #69100, #19524, #62740, .T. ) ;
#8058=DIRECTION ( 'NONE',  ( 0.000000000000000000, 0.000000000000000000, 1.000000000000000000 ) ) ;
#8059=VECTOR ( 'NONE', #55363, 1000.000000000000000 ) ;
#8131=( LENGTH_UNIT ( ) NAMED_UNIT ( * ) SI_UNIT ( .MILLI., .METRE. ) );
#8136=B_SPLINE_CURVE_WITH_KNOTS ( 'NONE', 3,
 ( #79110, #17759, #52243, #37765, #16871, #16428, #72728, #44550, #44104, #38637, #51806, #9604, #10496, #52682, #3247, #80005, #71840, #3682, #37314, #58629, #45436, #80442, #73159, #31822, #18198 ),
 .UNSPECIFIED., .F., .F.,
 ( 4, 2, 2, 2, 2, 2, 2, 2, 2, 1, 2, 2, 4 ),
 ( 0.05960644416065473405, 0.06208808443815339029, 0.06332890457690272534, 0.06456972471565204652, 0.06705136499315070275, 0.06829218513190002393, 0.06953300527064934511, 0.07201464554814800134, 0.07325546568689735027, 0.07449628582564669921, 0.07573710596439604814, 0.07697792610314539707, 0.07945956638064405331 ),
 .UNSPECIFIED. ) ;
#8139=CARTESIAN_POINT ( 'NONE',  ( -75.89055769641095139, 54.33720168335926815, 30.80247753283806844 ) ) ;
#8179=ORIENTED_EDGE ( 'NONE', *, *, #72960, .F. ) ;
#8196=VECTOR ( 'NONE', #66336, 1000.000000000000114 ) ;
#8230=CARTESIAN_POINT ( 'NONE',  ( -47.82553099389205187, 100.8041302358256814, 75.75399279458846991 ) ) ;
#8232=DIRECTION ( 'NONE',  ( 1.000000000000000000, 0.000000000000000000, 0.000000000000000000 ) ) ;
#8235=FACE_OUTER_BOUND ( 'NONE', #52359, .T. ) ;
#8238=ADVANCED_FACE ( 'NONE', ( #59039 ), #85459, .F. ) ;
#8246=DIRECTION ( 'NONE',  ( -0.000000000000000000, 1.000000000000000000, -0.000000000000000000 ) ) ;
#8329=DIRECTION ( 'NONE',  ( -0.000000000000000000, -1.000000000000000000, -0.000000000000000000 ) ) ;
#8364=ORIENTED_EDGE ( 'NONE', *, *, #80879, .T. ) ;
#8375=CARTESIAN_POINT ( 'NONE',  ( 61.00843881761244347, 65.60000000000000853, -33.74458626278666884 ) ) ;
#8382=ORIENTED_EDGE ( 'NONE', *, *, #8566, .T. ) ;
#8426=EDGE_LOOP ( 'NONE', ( #76762, #16841, #34066, #28559 ) ) ;
#8454=VECTOR ( 'NONE', #938, 1000.000000000000000 ) ;
#8470=VERTEX_POINT ( 'NONE', #21305 ) ;
#8482=ORIENTED_EDGE ( 'NONE', *, *, #35140, .T. ) ;
#8492=CARTESIAN_POINT ( 'NONE',  ( -546.0365000000000464, 53.97500000000000142, 50.79999999999999716 ) ) ;
#8498=CARTESIAN_POINT ( 'NONE',  ( -15.60269531711297830, 92.07499999999998863, -52.58204823848948450 ) ) ;
#8502=DIRECTION ( 'NONE',  ( -1.000000000000000000, 0.000000000000000000, 0.000000000000000000 ) ) ;
#8537=CARTESIAN_POINT ( 'NONE',  ( -487.2989999999999782, 6.038608028953049711, 90.48749999999999716 ) ) ;
#8550=VECTOR ( 'NONE', #6730, 1000.000000000000000 ) ;
#8566=EDGE_CURVE ( 'NONE', #16628, #88630, #35815, .T. ) ;
#8586=AXIS2_PLACEMENT_3D ( 'NONE', #45884, #66800, #11848 ) ;
#8595=COLOUR_RGB ( '', 0.31764706, 0.68627451, 0.89019608) ;
#8613=CARTESIAN_POINT ( 'NONE',  ( -487.2989999999999782, 100.8062500000000057, 94.61194598552329182 ) ) ;
#8624=DIRECTION ( 'NONE',  ( -1.000000000000000000, 0.000000000000000000, 0.000000000000000000 ) ) ;
#8650=ORIENTED_EDGE ( 'NONE', *, *, #22790, .T. ) ;
#8664=ORIENTED_EDGE ( 'NONE', *, *, #38112, .F. ) ;
#8670=CARTESIAN_POINT ( 'NONE',  ( -2.852988951225258196E-12, 11.69999999999217977, 8.005813272589510943E-12 ) ) ;
#8676=ORIENTED_EDGE ( 'NONE', *, *, #55628, .T. ) ;
#8683=CARTESIAN_POINT ( 'NONE',  ( -12.51828503297007167, 80.89413879163728893, 117.6922344853366127 ) ) ;
#8684=ORIENTED_EDGE ( 'NONE', *, *, #280, .F. ) ;
#8696=CARTESIAN_POINT ( 'NONE',  ( -487.2989999999999782, 22.53639197104660141, 90.48749999999999716 ) ) ;
#8697=EDGE_CURVE ( 'NONE', #59609, #24211, #79420, .T. ) ;
#8698=VERTEX_POINT ( 'NONE', #84894 ) ;
#8722=CARTESIAN_POINT ( 'NONE',  ( -458.3598257906459708, 47.62500000000000000, 3.174999999999999822 ) ) ;
#8728=CARTESIAN_POINT ( 'NONE',  ( 11.48301363694224442, 87.75296475977089017, 117.7977433391754118 ) ) ;
#8781=CARTESIAN_POINT ( 'NONE',  ( -487.2989999999999782, 101.9113919710471947, 11.11250000000054072 ) ) ;
#8809=VERTEX_POINT ( 'NONE', #42022 ) ;
#8819=CARTESIAN_POINT ( 'NONE',  ( 0.000000000000000000, 101.5999999999999943, 0.000000000000000000 ) ) ;
#8820=DIRECTION ( 'NONE',  ( 0.000000000000000000, 0.000000000000000000, -1.000000000000000000 ) ) ;
#8826=AXIS2_PLACEMENT_3D ( 'NONE', #80781, #60302, #11270 ) ;
#8832=DIRECTION ( 'NONE',  ( 0.000000000000000000, 0.000000000000000000, 1.000000000000000000 ) ) ;
#8843=DIRECTION ( 'NONE',  ( 0.000000000000000000, 1.000000000000000000, 0.000000000000000000 ) ) ;
#8847=ADVANCED_FACE ( 'NONE', ( #77015 ), #77914, .T. ) ;
#8859=VERTEX_POINT ( 'NONE', #49735 ) ;
#8878=AXIS2_PLACEMENT_3D ( 'NONE', #39164, #40051, #19615 ) ;
#8895=CARTESIAN_POINT ( 'NONE',  ( 0.000000000000000000, 100.5999999999999659, 0.000000000000000000 ) ) ;
#8932=DIRECTION ( 'NONE',  ( 0.000000000000000000, 0.000000000000000000, -1.000000000000000000 ) ) ;
#8958=DIRECTION ( 'NONE',  ( -0.000000000000000000, 1.000000000000000000, -0.000000000000000000 ) ) ;
#8974=TOROIDAL_SURFACE ( 'NONE', #87291, 36.57600000000000051, 1.524000000000000021 ) ;
#8989=PLANE ( 'NONE',  #69429 ) ;
#9018=DIRECTION ( 'NONE',  ( 0.9586846635221889512, 0.000000000000000000, -0.2844709403917162205 ) ) ;
#9022=VERTEX_POINT ( 'NONE', #33819 ) ;
#9029=EDGE_CURVE ( 'NONE', #74702, #47878, #46532, .T. ) ;
#9036=ORIENTED_EDGE ( 'NONE', *, *, #30296, .F. ) ;
#9039=AXIS2_PLACEMENT_3D ( 'NONE', #9867, #72095, #31183 ) ;
#9041=LINE ( 'NONE', #48986, #46279 ) ;
#9055=EDGE_CURVE ( 'NONE', #65784, #88397, #42900, .T. ) ;
#9069=DIRECTION ( 'NONE',  ( 0.000000000000000000, 0.000000000000000000, 1.000000000000000000 ) ) ;
#9074=DIRECTION ( 'NONE',  ( 0.000000000000000000, 1.000000000000000000, 0.000000000000000000 ) ) ;
#9125=CARTESIAN_POINT ( 'NONE',  ( 70.63919639214310564, 65.60000000000000853, -53.97512327982435210 ) ) ;
#9141=CARTESIAN_POINT ( 'NONE',  ( -446.0240000000000009, 93.66249999999999432, 90.48749999999999716 ) ) ;
#9149=CARTESIAN_POINT ( 'NONE',  ( -446.0240000000000009, 3.174999999999999822, 50.79999999999999716 ) ) ;
#9152=ORIENTED_EDGE ( 'NONE', *, *, #21504, .F. ) ;
#9175=CARTESIAN_POINT ( 'NONE',  ( 10.01454489833087003, 74.85873851776135268, 117.9324610216481517 ) ) ;
#9194=EDGE_CURVE ( 'NONE', #71111, #35866, #73358, .T. ) ;
#9195=DIRECTION ( 'NONE',  ( 0.000000000000000000, 1.047445008332813989E-14, -1.000000000000000000 ) ) ;
#9248=VECTOR ( 'NONE', #82071, 1000.000000000000000 ) ;
#9259=ORIENTED_EDGE ( 'NONE', *, *, #65988, .F. ) ;
#9267=DIRECTION ( 'NONE',  ( 1.000000000000000000, 0.000000000000000000, 0.000000000000000000 ) ) ;
#9285=CARTESIAN_POINT ( 'NONE',  ( 69.63919639214310564, 101.5999999999999943, 56.85413200336908801 ) ) ;
#9288=VERTEX_POINT ( 'NONE', #66427 ) ;
#9293=CARTESIAN_POINT ( 'NONE',  ( -487.2989999999999782, 6.038608028953049711, 90.48749999999999716 ) ) ;
#9334=PLANE ( 'NONE',  #53141 ) ;
#9398=CARTESIAN_POINT ( 'NONE',  ( -41.60202597009397607, 76.06518036156089124, 47.15338361873602935 ) ) ;
#9408=ORIENTED_EDGE ( 'NONE', *, *, #13796, .F. ) ;
#9414=CARTESIAN_POINT ( 'NONE',  ( -546.0365000000000464, 53.97500000000000142, 50.79999999999999716 ) ) ;
#9419=FACE_OUTER_BOUND ( 'NONE', #77322, .T. ) ;
#9424=AXIS2_PLACEMENT_3D ( 'NONE', #65659, #59285, #52006 ) ;
#9435=DIRECTION ( 'NONE',  ( -1.000000000000000000, 0.000000000000000000, 0.000000000000000000 ) ) ;
#9445=CARTESIAN_POINT ( 'NONE',  ( -469.3583484187089994, 53.97500000000000142, -3.174999999999999822 ) ) ;
#9452=DIRECTION ( 'NONE',  ( 0.000000000000000000, 0.000000000000000000, -1.000000000000000000 ) ) ;
#9485=AXIS2_PLACEMENT_3D ( 'NONE', #31684, #59381, #25318 ) ;
#9520=EDGE_CURVE ( 'NONE', #7908, #81729, #1883, .T. ) ;
#9534=VECTOR ( 'NONE', #89496, 1000.000000000000000 ) ;
#9541=DIRECTION ( 'NONE',  ( 0.000000000000000000, 0.000000000000000000, 1.000000000000000000 ) ) ;
#9593=ORIENTED_EDGE ( 'NONE', *, *, #36997, .F. ) ;
#9604=CARTESIAN_POINT ( 'NONE',  ( 8.377092249087933595, 92.10453133679206417, 118.2601133684811856 ) ) ;
#9631=VECTOR ( 'NONE', #18232, 1000.000000000000000 ) ;
#9681=CYLINDRICAL_SURFACE ( 'NONE', #1199, 118.5560000000000116 ) ;
#9686=ORIENTED_EDGE ( 'NONE', *, *, #64270, .T. ) ;
#9704=AXIS2_PLACEMENT_3D ( 'NONE', #23520, #17134, #3058 ) ;
#9712=CARTESIAN_POINT ( 'NONE',  ( -12.05184559704344593, 78.45907740360294724, 117.9422764726210602 ) ) ;
#9741=AXIS2_PLACEMENT_3D ( 'NONE', #35243, #61599, #6215 ) ;
#9752=ORIENTED_EDGE ( 'NONE', *, *, #38767, .T. ) ;
#9773=DIRECTION ( 'NONE',  ( 0.000000000000000000, -0.5000000000000061062, 0.8660254037844351549 ) ) ;
#9814=ORIENTED_EDGE ( 'NONE', *, *, #89251, .T. ) ;
#9826=DIRECTION ( 'NONE',  ( 0.7071067811865561215, 1.189321603860061305E-16, -0.7071067811865389130 ) ) ;
#9842=EDGE_LOOP ( 'NONE', ( #26792, #47677, #68908, #15386, #47022, #11163 ) ) ;
#9849=DIRECTION ( 'NONE',  ( -0.000000000000000000, -1.000000000000000000, -0.000000000000000000 ) ) ;
#9867=CARTESIAN_POINT ( 'NONE',  ( -544.5124999999999318, 53.97500000000000142, 14.22400000000000020 ) ) ;
#9875=PLANE ( 'NONE',  #11303 ) ;
#9909=ORIENTED_EDGE ( 'NONE', *, *, #75396, .F. ) ;
#9934=CARTESIAN_POINT ( 'NONE',  ( -492.0614999999999668, 14.28750000000026077, 11.11249999999970051 ) ) ;
#9953=AXIS2_PLACEMENT_3D ( 'NONE', #48779, #14294, #50128 ) ;
#9959=EDGE_CURVE ( 'NONE', #74494, #10702, #5001, .T. ) ;
#9987=DIRECTION ( 'NONE',  ( 0.000000000000000000, 1.000000000000000000, 0.000000000000000000 ) ) ;
#10009=VERTEX_POINT ( 'NONE', #87672 ) ;
#10029=DIRECTION ( 'NONE',  ( -0.000000000000000000, 1.000000000000000000, -0.000000000000000000 ) ) ;
#10051=CARTESIAN_POINT ( 'NONE',  ( -254.0000000000000000, 93.66249999999999432, 90.48749999999999716 ) ) ;
#10057=FACE_BOUND ( 'NONE', #73819, .T. ) ;
#10088=EDGE_CURVE ( 'NONE', #52469, #64816, #83906, .T. ) ;
#10119=FACE_OUTER_BOUND ( 'NONE', #66222, .T. ) ;
#10158=CARTESIAN_POINT ( 'NONE',  ( -8.388013673212871169, 72.97744838846872995, 118.2603890449115340 ) ) ;
#10159=CARTESIAN_POINT ( 'NONE',  ( -254.0000000000000000, 3.174999999999999822, 50.79999999999999716 ) ) ;
#10163=ORIENTED_EDGE ( 'NONE', *, *, #48411, .F. ) ;
#10170=( BOUNDED_CURVE ( )  B_SPLINE_CURVE ( 3, ( #82205, #88563, #13586, #19061 ),
 .UNSPECIFIED., .F., .T. ) 
 B_SPLINE_CURVE_WITH_KNOTS ( ( 4, 4 ),
 ( 1.719776299252462559, 1.732437064411955996 ),
 .UNSPECIFIED. ) 
 CURVE ( )  GEOMETRIC_REPRESENTATION_ITEM ( )  RATIONAL_B_SPLINE_CURVE ( ( 1.000000000000000000, 0.9999866421300730446, 0.9999866421300730446, 1.000000000000000000 ) ) 
 REPRESENTATION_ITEM ( '' )  );
#10232=CARTESIAN_POINT ( 'NONE',  ( -492.0614999999999668, 93.66249999999999432, 11.11250000000040217 ) ) ;
#10265=CIRCLE ( 'NONE', #43574, 4.762499999999999289 ) ;
#10276=AXIS2_PLACEMENT_3D ( 'NONE', #30965, #64160, #30080 ) ;
#10282=ORIENTED_EDGE ( 'NONE', *, *, #76853, .T. ) ;
#10321=ADVANCED_FACE ( 'NONE', ( #25223 ), #58404, .F. ) ;
#10338=ORIENTED_EDGE ( 'NONE', *, *, #15746, .T. ) ;
#10455=DIRECTION ( 'NONE',  ( -0.000000000000000000, 1.000000000000000000, -0.000000000000000000 ) ) ;
#10467=DIRECTION ( 'NONE',  ( 0.000000000000000000, -1.000000000000000000, 0.000000000000000000 ) ) ;
#10494=EDGE_LOOP ( 'NONE', ( #50510, #34195, #31839, #72704, #2096 ) ) ;
#10496=CARTESIAN_POINT ( 'NONE',  ( 8.684762001849648527, 91.82556179790852013, 118.2378372707471641 ) ) ;
#10519=CARTESIAN_POINT ( 'NONE',  ( -254.0000000000000000, 14.28749999999982201, 90.48749999999999716 ) ) ;
#10555=LINE ( 'NONE', #65956, #36154 ) ;
#10593=CARTESIAN_POINT ( 'NONE',  ( -2.077948353448777485, 70.01426914847409932, 118.5384880737505995 ) ) ;
#10614=EDGE_CURVE ( 'NONE', #72800, #40087, #16092, .T. ) ;
#10670=DIRECTION ( 'NONE',  ( 1.000000000000000000, 0.000000000000000000, 0.000000000000000000 ) ) ;
#10687=VERTEX_POINT ( 'NONE', #8375 ) ;
#10694=FACE_OUTER_BOUND ( 'NONE', #3683, .T. ) ;
#10702=VERTEX_POINT ( 'NONE', #14297 ) ;
#10712=DIRECTION ( 'NONE',  ( -0.2884130866282269556, 0.7071067811865447972, 0.6456143519637576045 ) ) ;
#10751=AXIS2_PLACEMENT_3D ( 'NONE', #6511, #41459, #69187 ) ;
#10760=CARTESIAN_POINT ( 'NONE',  ( -465.6921742093550165, 47.62500000000000000, 3.174999999999999822 ) ) ;
#10762=CARTESIAN_POINT ( 'NONE',  ( 70.63919639214310564, 49.07499999999999574, -53.97512327982435210 ) ) ;
#10778=EDGE_CURVE ( 'NONE', #52534, #17788, #87796, .T. ) ;
#10787=CARTESIAN_POINT ( 'NONE',  ( -492.0614999999999668, 14.28749999999982201, 85.72499999999999432 ) ) ;
#10788=CARTESIAN_POINT ( 'NONE',  ( -40.89999999999999858, 53.97500000000000142, 30.79999999999999361 ) ) ;
#10819=CARTESIAN_POINT ( 'NONE',  ( -462.0260000000000105, 53.97500000000000142, -1.387778780781445991E-14 ) ) ;
#10848=EDGE_CURVE ( 'NONE', #34776, #76744, #60980, .T. ) ;
#10862=EDGE_LOOP ( 'NONE', ( #89859, #72958 ) ) ;
#10887=AXIS2_PLACEMENT_3D ( 'NONE', #63416, #1198, #28908 ) ;
#10895=ORIENTED_EDGE ( 'NONE', *, *, #60157, .T. ) ;
#10897=CARTESIAN_POINT ( 'NONE',  ( -479.3614999999999782, 3.174999999999999822, -1.387778780781445991E-14 ) ) ;
#10925=ADVANCED_FACE ( 'NONE', ( #20555 ), #75958, .F. ) ;
#10945=VERTEX_POINT ( 'NONE', #48670 ) ;
#10966=VERTEX_POINT ( 'NONE', #8722 ) ;
#10992=CARTESIAN_POINT ( 'NONE',  ( -479.3614999999999782, 21.43125000000029701, 15.23694598552314972 ) ) ;
#11014=FACE_BOUND ( 'NONE', #2325, .T. ) ;
#11032=LINE ( 'NONE', #52334, #45761 ) ;
#11036=VECTOR ( 'NONE', #81006, 1000.000000000000000 ) ;
#11037=DIRECTION ( 'NONE',  ( 0.7071067811865573427, -0.7071067811865376918, 1.287852911526298168E-16 ) ) ;
#11042=DIRECTION ( 'NONE',  ( -1.000000000000000000, 0.000000000000000000, 0.000000000000000000 ) ) ;
#11067=CARTESIAN_POINT ( 'NONE',  ( -47.02966122971777452, 101.5999999999999943, 107.7386843274874053 ) ) ;
#11070=CARTESIAN_POINT ( 'NONE',  ( -0.8023776826656670025, 65.59999999999998010, -4.197052493943455254 ) ) ;
#11086=CARTESIAN_POINT ( 'NONE',  ( -479.3614999999999782, 93.66249999999999432, 82.23860802895320887 ) ) ;
#11131=CARTESIAN_POINT ( 'NONE',  ( -487.2989999999999782, 97.78694598552380057, 3.968750000000479616 ) ) ;
#11139=FACE_OUTER_BOUND ( 'NONE', #63943, .T. ) ;
#11150=ORIENTED_EDGE ( 'NONE', *, *, #54100, .T. ) ;
#11162=CARTESIAN_POINT ( 'NONE',  ( -487.2989999999999782, 89.53805401447691281, 18.25625000000039933 ) ) ;
#11163=ORIENTED_EDGE ( 'NONE', *, *, #925, .F. ) ;
#11164=PRODUCT ( 'Rotary Table Drive Mechanism', 'Rotary Table Drive Mechanism', '', ( #74016 ) ) ;
#11169=AXIS2_PLACEMENT_3D ( 'NONE', #51579, #65665, #45209 ) ;
#11211=VERTEX_POINT ( 'NONE', #23694 ) ;
#11225=DIRECTION ( 'NONE',  ( 0.8861241255175467124, 0.000000000000000000, -0.4634479843259253218 ) ) ;
#11233=VERTEX_POINT ( 'NONE', #2346 ) ;
#11248=VECTOR ( 'NONE', #80317, 1000.000000000000114 ) ;
#11270=DIRECTION ( 'NONE',  ( 0.000000000000000000, -1.000000000000000000, -8.792068030499130893E-15 ) ) ;
#11300=CIRCLE ( 'NONE', #22938, 17.33514202138210081 ) ;
#11303=AXIS2_PLACEMENT_3D ( 'NONE', #33436, #5292, #39786 ) ;
#11304=LINE ( 'NONE', #66716, #4191 ) ;
#11312=CARTESIAN_POINT ( 'NONE',  ( -479.3614999999999782, 18.41194598552320016, 97.63125000000000853 ) ) ;
#11342=EDGE_CURVE ( 'NONE', #64560, #53581, #64940, .T. ) ;
#11380=CARTESIAN_POINT ( 'NONE',  ( -48.67264380398864176, 148.4450814996825443, 66.68100227564391957 ) ) ;
#11396=VECTOR ( 'NONE', #48569, 1000.000000000000114 ) ;
#11397=AXIS2_PLACEMENT_3D ( 'NONE', #18514, #89367, #74836 ) ;
#11405=ORIENTED_EDGE ( 'NONE', *, *, #40947, .F. ) ;
#11415=DIRECTION ( 'NONE',  ( 0.000000000000000000, 0.000000000000000000, -1.000000000000000000 ) ) ;
#11441=AXIS2_PLACEMENT_3D ( 'NONE', #82081, #19829, #13464 ) ;
#11464=LINE ( 'NONE', #40504, #66774 ) ;
#11466=CARTESIAN_POINT ( 'NONE',  ( -17.54031676229692849, 65.59999999999998010, 43.71138335376673467 ) ) ;
#11473=CARTESIAN_POINT ( 'NONE',  ( -487.2989999999999782, 21.43125000000029701, 15.23694598552314972 ) ) ;
#11493=LINE ( 'NONE', #45982, #63809 ) ;
#11497=CARTESIAN_POINT ( 'NONE',  ( -487.2989999999999782, 93.66249999999999432, 98.73639197104678544 ) ) ;
#11511=CARTESIAN_POINT ( 'NONE',  ( -12.60000000000000142, 82.54999999999999716, 117.6834004267381744 ) ) ;
#11544=CARTESIAN_POINT ( 'NONE',  ( -479.3614999999999782, 53.97500000000000142, 12.69999999999999929 ) ) ;
#11561=DIRECTION ( 'NONE',  ( -0.000000000000000000, 1.000000000000000000, -0.000000000000000000 ) ) ;
#11583=CARTESIAN_POINT ( 'NONE',  ( -41.60202597009397607, 64.60000000000000853, 50.85338361873603219 ) ) ;
#11600=EDGE_CURVE ( 'NONE', #67868, #77207, #71286, .T. ) ;
#11609=DIRECTION ( 'NONE',  ( 0.000000000000000000, 7.536132396315209176E-17, -1.000000000000000000 ) ) ;
#11622=FACE_OUTER_BOUND ( 'NONE', #62923, .T. ) ;
#11631=ORIENTED_EDGE ( 'NONE', *, *, #64470, .T. ) ;
#11655=EDGE_LOOP ( 'NONE', ( #40444, #75966, #81341, #83460 ) ) ;
#11656=EDGE_CURVE ( 'NONE', #53776, #41996, #24464, .T. ) ;
#11667=DIRECTION ( 'NONE',  ( -1.000000000000000000, 0.000000000000000000, 0.000000000000000000 ) ) ;
#11695=VECTOR ( 'NONE', #14565, 1000.000000000000114 ) ;
#11727=CARTESIAN_POINT ( 'NONE',  ( -11.39789362727886157, 88.16700649416421243, 118.0069991474212259 ) ) ;
#11733=ORIENTED_EDGE ( 'NONE', *, *, #78019, .F. ) ;
#11738=DIRECTION ( 'NONE',  ( 0.000000000000000000, 0.8660254037844379305, 0.5000000000000011102 ) ) ;
#11765=CARTESIAN_POINT ( 'NONE',  ( -48.02966122971777452, 100.5999999999999659, 106.4272185163641780 ) ) ;
#11770=CARTESIAN_POINT ( 'NONE',  ( 69.63919639214307722, 92.07499999999998863, 0.000000000000000000 ) ) ;
#11785=ORIENTED_EDGE ( 'NONE', *, *, #56860, .T. ) ;
#11788=VERTEX_POINT ( 'NONE', #52571 ) ;
#11802=DIRECTION ( 'NONE',  ( 1.000000000000000000, 0.000000000000000000, 0.000000000000000000 ) ) ;
#11832=CARTESIAN_POINT ( 'NONE',  ( -41.60202597009397607, 64.60000000000000853, 50.85338361873603219 ) ) ;
#11848=DIRECTION ( 'NONE',  ( 0.000000000000000000, 0.5000000000000087708, -0.8660254037844334896 ) ) ;
#11851=CARTESIAN_POINT ( 'NONE',  ( 0.000000000000000000, 65.60000000000000853, -53.97512327982435210 ) ) ;
#11867=CIRCLE ( 'NONE', #85874, 4.762500000000001066 ) ;
#11914=DIRECTION ( 'NONE',  ( 0.000000000000000000, 1.000000000000000000, 0.000000000000000000 ) ) ;
#11916=CARTESIAN_POINT ( 'NONE',  ( 50.42303506447345285, 65.60000000000000853, -73.21698938693724301 ) ) ;
#11946=CARTESIAN_POINT ( 'NONE',  ( 61.00843881761244347, 49.07499999999999574, -53.97512327982435210 ) ) ;
#11980=DIRECTION ( 'NONE',  ( 1.000000000000000000, 0.000000000000000000, 0.000000000000000000 ) ) ;
#12039=CARTESIAN_POINT ( 'NONE',  ( -492.0614999999999668, 93.66249999999999432, 85.72499999999999432 ) ) ;
#12096=ORIENTED_EDGE ( 'NONE', *, *, #36867, .T. ) ;
#12161=CIRCLE ( 'NONE', #77452, 87.89999999999994884 ) ;
#12165=CARTESIAN_POINT ( 'NONE',  ( -41.60202597009397607, 40.59999999999997300, 47.15338361873602935 ) ) ;
#12166=ORIENTED_EDGE ( 'NONE', *, *, #64270, .F. ) ;
#12169=B_SPLINE_CURVE_WITH_KNOTS ( 'NONE', 3,
 ( #67831, #86503, #45133, #38330 ),
 .UNSPECIFIED., .F., .F.,
 ( 4, 4 ),
 ( 0.000000000000000000, 0.001501537230210108625 ),
 .UNSPECIFIED. ) ;
#12182=VERTEX_POINT ( 'NONE', #14194 ) ;
#12225=DIRECTION ( 'NONE',  ( 1.000000000000000000, 0.000000000000000000, 0.000000000000000000 ) ) ;
#12227=CARTESIAN_POINT ( 'NONE',  ( 70.63919639214310564, 353.0471713899363522, 56.85413200336923012 ) ) ;
#12264=CARTESIAN_POINT ( 'NONE',  ( 0.000000000000000000, 65.60000000000000853, 118.5560000000000116 ) ) ;
#12307=CARTESIAN_POINT ( 'NONE',  ( 12.60000000000000142, 82.54999999999999716, 89.46299999999996544 ) ) ;
#12311=DIRECTION ( 'NONE',  ( 0.000000000000000000, -1.000000000000000000, -2.913971193241881161E-15 ) ) ;
#12332=VERTEX_POINT ( 'NONE', #77317 ) ;
#12352=DIRECTION ( 'NONE',  ( 0.000000000000000000, 0.000000000000000000, 1.000000000000000000 ) ) ;
#12366=LINE ( 'NONE', #67774, #41389 ) ;
#12377=ORIENTED_EDGE ( 'NONE', *, *, #56017, .T. ) ;
#12384=AXIS2_PLACEMENT_3D ( 'NONE', #50089, #41927, #7877 ) ;
#12411=DIRECTION ( 'NONE',  ( 0.9586846635221889512, 0.000000000000000000, -0.2844709403917162205 ) ) ;
#12423=PLANE ( 'NONE',  #28488 ) ;
#12436=EDGE_LOOP ( 'NONE', ( #74058, #58884, #77020, #26816 ) ) ;
#12442=EDGE_LOOP ( 'NONE', ( #18103, #71966, #76608, #40160 ) ) ;
#12445=CARTESIAN_POINT ( 'NONE',  ( -17.13243906362141900, 64.60000000000000853, 42.79834678115690849 ) ) ;
#12450=EDGE_CURVE ( 'NONE', #22374, #30549, #48983, .T. ) ;
#12502=CARTESIAN_POINT ( 'NONE',  ( -55.95243198108136085, 55.97500000000000142, 70.69974874213239957 ) ) ;
#12510=ORIENTED_EDGE ( 'NONE', *, *, #49148, .T. ) ;
#12511=EDGE_CURVE ( 'NONE', #74649, #30366, #66802, .T. ) ;
#12523=ORIENTED_EDGE ( 'NONE', *, *, #22939, .T. ) ;
#12552=ORIENTED_EDGE ( 'NONE', *, *, #3450, .T. ) ;
#12566=CARTESIAN_POINT ( 'NONE',  ( -462.0260000000000105, 53.97500000000000142, -3.174999999999999822 ) ) ;
#12576=EDGE_CURVE ( 'NONE', #87213, #6718, #80911, .T. ) ;
#12591=ORIENTED_EDGE ( 'NONE', *, *, #73202, .T. ) ;
#12603=ORIENTED_EDGE ( 'NONE', *, *, #56028, .F. ) ;
#12607=AXIS2_PLACEMENT_3D ( 'NONE', #15319, #8958, #30722 ) ;
#12608=DIRECTION ( 'NONE',  ( -1.000000000000000000, 0.000000000000000000, 0.000000000000000000 ) ) ;
#12642=ORIENTED_EDGE ( 'NONE', *, *, #26714, .F. ) ;
#12645=ORIENTED_EDGE ( 'NONE', *, *, #44877, .T. ) ;
#12658=EDGE_CURVE ( 'NONE', #76744, #17700, #5032, .T. ) ;
#12661=DIRECTION ( 'NONE',  ( -0.000000000000000000, 1.000000000000000000, -0.000000000000000000 ) ) ;
#12669=EDGE_CURVE ( 'NONE', #877, #19584, #13636, .T. ) ;
#12677=ORIENTED_EDGE ( 'NONE', *, *, #40616, .T. ) ;
#12687=ORIENTED_EDGE ( 'NONE', *, *, #75604, .F. ) ;
#12688=DIRECTION ( 'NONE',  ( -1.000000000000000000, 0.000000000000000000, 0.000000000000000000 ) ) ;
#12705=FACE_BOUND ( 'NONE', #29529, .T. ) ;
#12723=VECTOR ( 'NONE', #66144, 1000.000000000000000 ) ;
#12773=AXIS2_PLACEMENT_3D ( 'NONE', #83599, #47251, #26820 ) ;
#12776=ORIENTED_EDGE ( 'NONE', *, *, #58820, .T. ) ;
#12798=B_SPLINE_CURVE_WITH_KNOTS ( 'NONE', 3,
 ( #53580, #18646, #39975, #25457 ),
 .UNSPECIFIED., .F., .F.,
 ( 4, 4 ),
 ( 0.000000000000000000, 0.001454366796625762874 ),
 .UNSPECIFIED. ) ;
#12812=VECTOR ( 'NONE', #24579, 999.9999999999998863 ) ;
#12848=EDGE_CURVE ( 'NONE', #78132, #21144, #36631, .T. ) ;
#12857=VECTOR ( 'NONE', #13900, 1000.000000000000000 ) ;
#12862=CIRCLE ( 'NONE', #66532, 4.762500000000002842 ) ;
#12872=DIRECTION ( 'NONE',  ( -1.000000000000000000, 0.000000000000000000, 0.000000000000000000 ) ) ;
#12884=EDGE_LOOP ( 'NONE', ( #60433, #2226, #21209, #83447 ) ) ;
#12927=CARTESIAN_POINT ( 'NONE',  ( -462.0260000000000105, 53.97500000000000142, -3.174999999999999822 ) ) ;
#12963=LINE ( 'NONE', #40652, #42983 ) ;
#12986=ORIENTED_EDGE ( 'NONE', *, *, #49151, .T. ) ;
#12988=LINE ( 'NONE', #62906, #59399 ) ;
#12997=PLANE ( 'NONE',  #17684 ) ;
#13017=DIRECTION ( 'NONE',  ( 1.000000000000000000, 0.000000000000000000, 0.000000000000000000 ) ) ;
#13026=LINE ( 'NONE', #7101, #70918 ) ;
#13033=CARTESIAN_POINT ( 'NONE',  ( -41.60202597009397607, 40.59999999999997300, 54.66767516814134353 ) ) ;
#13052=VERTEX_POINT ( 'NONE', #72484 ) ;
#13054=VECTOR ( 'NONE', #88419, 1000.000000000000000 ) ;
#13083=LINE ( 'NONE', #87151, #85251 ) ;
#13101=ORIENTED_EDGE ( 'NONE', *, *, #23588, .F. ) ;
#13105=DIRECTION ( 'NONE',  ( -0.8660254037844351549, 0.5000000000000061062, 0.000000000000000000 ) ) ;
#13127=ORIENTED_EDGE ( 'NONE', *, *, #65988, .T. ) ;
#13145=AXIS2_PLACEMENT_3D ( 'NONE', #8781, #35112, #1516 ) ;
#13152=DIRECTION ( 'NONE',  ( 0.000000000000000000, 0.000000000000000000, -1.000000000000000000 ) ) ;
#13158=CARTESIAN_POINT ( 'NONE',  ( -254.0000000000000000, 3.174999999999999822, -41.27499999999999858 ) ) ;
#13203=ORIENTED_EDGE ( 'NONE', *, *, #22035, .F. ) ;
#13220=CIRCLE ( 'NONE', #49639, 4.762500000000000178 ) ;
#13234=CIRCLE ( 'NONE', #194, 3.814291549405317117 ) ;
#13237=LINE ( 'NONE', #54085, #37812 ) ;
#13253=DIRECTION ( 'NONE',  ( 0.9329458799396118662, 0.000000000000000000, -0.3600166455925385423 ) ) ;
#13263=EDGE_LOOP ( 'NONE', ( #48150, #2153 ) ) ;
#13316=CARTESIAN_POINT ( 'NONE',  ( -479.3614999999999782, 86.51875000000001137, 94.61194598552339130 ) ) ;
#13335=ORIENTED_EDGE ( 'NONE', *, *, #31363, .T. ) ;
#13383=CARTESIAN_POINT ( 'NONE',  ( -47.04228170325576031, 92.15829462204605704, 74.35109477667292310 ) ) ;
#13441=VERTEX_POINT ( 'NONE', #9149 ) ;
#13454=CARTESIAN_POINT ( 'NONE',  ( -465.6921742093550165, 47.62500000000000000, 3.174999999999999822 ) ) ;
#13464=DIRECTION ( 'NONE',  ( 0.000000000000000000, 1.000000000000000000, 0.000000000000000000 ) ) ;
#13496=DIRECTION ( 'NONE',  ( 0.000000000000000000, 0.000000000000000000, -1.000000000000000000 ) ) ;
#13500=CARTESIAN_POINT ( 'NONE',  ( -546.0365000000000464, 53.97500000000000142, 12.69999999999999929 ) ) ;
#13554=CARTESIAN_POINT ( 'NONE',  ( 69.39078715552076915, 92.39984138453077378, 54.48432155457955162 ) ) ;
#13564=DIRECTION ( 'NONE',  ( 1.000000000000000000, 0.000000000000000000, 0.000000000000000000 ) ) ;
#13570=CYLINDRICAL_SURFACE ( 'NONE', #87157, 4.762500000000001066 ) ;
#13573=DIRECTION ( 'NONE',  ( 0.000000000000000000, 1.000000000000000000, -0.000000000000000000 ) ) ;
#13586=CARTESIAN_POINT ( 'NONE',  ( -47.13180528695278326, 100.9330007194059675, 75.77065372412548072 ) ) ;
#13636=LINE ( 'NONE', #20011, #5008 ) ;
#13691=CARTESIAN_POINT ( 'NONE',  ( -462.0260000000000105, 53.97500000000000142, -3.174999999999999822 ) ) ;
#13710=VECTOR ( 'NONE', #86534, 1000.000000000000000 ) ;
#13755=DIRECTION ( 'NONE',  ( 0.000000000000000000, -1.000000000000000000, 0.000000000000000000 ) ) ;
#13760=ORIENTED_EDGE ( 'NONE', *, *, #49151, .F. ) ;
#13789=ADVANCED_FACE ( 'NONE', ( #48101 ), #63091, .T. ) ;
#13792=CARTESIAN_POINT ( 'NONE',  ( -487.2989999999999782, 93.66249999999999432, 90.48749999999999716 ) ) ;
#13796=EDGE_CURVE ( 'NONE', #19, #26777, #35379, .T. ) ;
#13900=DIRECTION ( 'NONE',  ( 0.000000000000000000, 0.000000000000000000, 1.000000000000000000 ) ) ;
#13910=EDGE_CURVE ( 'NONE', #19, #84869, #45645, .T. ) ;
#13912=FACE_BOUND ( 'NONE', #9842, .T. ) ;
#13927=ORIENTED_EDGE ( 'NONE', *, *, #64050, .T. ) ;
#13941=ORIENTED_EDGE ( 'NONE', *, *, #7988, .T. ) ;
#13949=DIRECTION ( 'NONE',  ( 0.000000000000000000, 1.000000000000000000, 0.000000000000000000 ) ) ;
#13961=AXIS2_PLACEMENT_3D ( 'NONE', #11832, #67232, #45871 ) ;
#13983=DIRECTION ( 'NONE',  ( 1.000000000000000000, -7.570719237730591757E-15, 0.000000000000000000 ) ) ;
#13991=EDGE_LOOP ( 'NONE', ( #15162, #31055, #55037, #24336 ) ) ;
#14009=ORIENTED_EDGE ( 'NONE', *, *, #59501, .F. ) ;
#14010=CARTESIAN_POINT ( 'NONE',  ( -47.02966122971772478, 92.07499999999998863, -43.25671021339634592 ) ) ;
#14023=CARTESIAN_POINT ( 'NONE',  ( -24.20305689751608824, 53.97499999999997300, 58.62596543806478877 ) ) ;
#14030=CIRCLE ( 'NONE', #64800, 4.762500000000002842 ) ;
#14031=ORIENTED_EDGE ( 'NONE', *, *, #78336, .F. ) ;
#14048=PLANE ( 'NONE',  #76076 ) ;
#14055=ORIENTED_EDGE ( 'NONE', *, *, #59325, .F. ) ;
#14090=DIRECTION ( 'NONE',  ( 1.000000000000000000, 0.000000000000000000, 0.000000000000000000 ) ) ;
#14098=DIRECTION ( 'NONE',  ( 0.000000000000000000, -0.5000000000000007772, 0.8660254037844381525 ) ) ;
#14144=EDGE_CURVE ( 'NONE', #21144, #55523, #75631, .T. ) ;
#14194=CARTESIAN_POINT ( 'NONE',  ( -487.2989999999999782, 89.53805401447691281, 18.25625000000039933 ) ) ;
#14203=DIRECTION ( 'NONE',  ( 0.000000000000000000, 0.000000000000000000, -1.000000000000000000 ) ) ;
#14208=VERTEX_POINT ( 'NONE', #56505 ) ;
#14231=ORIENTED_EDGE ( 'NONE', *, *, #88605, .F. ) ;
#14235=LINE ( 'NONE', #69643, #9248 ) ;
#14294=DIRECTION ( 'NONE',  ( 0.000000000000000000, 0.8660254037844445918, -0.4999999999999897304 ) ) ;
#14297=CARTESIAN_POINT ( 'NONE',  ( 0.000000000000000000, 100.5999999999999659, 118.5560000000000116 ) ) ;
#14354=AXIS2_PLACEMENT_3D ( 'NONE', #68709, #34168, #70052 ) ;
#14387=DIRECTION ( 'NONE',  ( 1.000000000000000000, -0.000000000000000000, -0.000000000000000000 ) ) ;
#14427=VECTOR ( 'NONE', #88622, 1000.000000000000000 ) ;
#14429=EDGE_CURVE ( 'NONE', #16194, #78995, #54511, .T. ) ;
#14441=ORIENTED_EDGE ( 'NONE', *, *, #2403, .F. ) ;
#14461=CARTESIAN_POINT ( 'NONE',  ( -462.0260000000000105, 53.97500000000000142, -1.387778780781445991E-14 ) ) ;
#14473=DIRECTION ( 'NONE',  ( 0.000000000000000000, 1.365923996832131856E-16, -1.000000000000000000 ) ) ;
#14474=VERTEX_POINT ( 'NONE', #60067 ) ;
#14565=DIRECTION ( 'NONE',  ( -0.5000000000000129896, -0.8660254037844311581, 0.000000000000000000 ) ) ;
#14597=CARTESIAN_POINT ( 'NONE',  ( 4.788368984666157546E-15, 92.07499999999998863, -39.10000000000005116 ) ) ;
#14599=VERTEX_POINT ( 'NONE', #46438 ) ;
#14600=CIRCLE ( 'NONE', #81328, 4.762500000000002842 ) ;
#14613=DIRECTION ( 'NONE',  ( 0.000000000000000000, 0.000000000000000000, -1.000000000000000000 ) ) ;
#14654=CARTESIAN_POINT ( 'NONE',  ( -2.861372676390278258, 94.82780855858955249, 118.3221063943049813 ) ) ;
#14674=ORIENTED_EDGE ( 'NONE', *, *, #21687, .T. ) ;
#14694=( NAMED_UNIT ( * ) SI_UNIT ( $, .STERADIAN. ) SOLID_ANGLE_UNIT ( ) );
#14699=CARTESIAN_POINT ( 'NONE',  ( -487.2989999999999782, 14.28750000000036025, 2.863608028952925100 ) ) ;
#14703=CARTESIAN_POINT ( 'NONE',  ( -479.3614999999999782, 53.97500000000000142, 88.90000000000000568 ) ) ;
#14721=LINE ( 'NONE', #56475, #33073 ) ;
#14754=ADVANCED_FACE ( 'NONE', ( #1459 ), #20558, .T. ) ;
#14839=EDGE_CURVE ( 'NONE', #877, #23402, #16868, .T. ) ;
#14847=EDGE_CURVE ( 'NONE', #33225, #16017, #2799, .T. ) ;
#14856=EDGE_LOOP ( 'NONE', ( #40368, #33154, #4123, #80140 ) ) ;
#14882=VERTEX_POINT ( 'NONE', #44996 ) ;
#14900=ORIENTED_EDGE ( 'NONE', *, *, #33359, .F. ) ;
#14935=EDGE_CURVE ( 'NONE', #53803, #53776, #47227, .T. ) ;
#14953=EDGE_CURVE ( 'NONE', #70548, #87213, #59957, .T. ) ;
#14954=SURFACE_STYLE_USAGE ( .BOTH. , #43526 ) ;
#14957=EDGE_CURVE ( 'NONE', #24976, #2162, #12798, .T. ) ;
#14961=CARTESIAN_POINT ( 'NONE',  ( -479.3614999999999782, 7.143750000000339995, 6.988054014476278830 ) ) ;
#14965=EDGE_LOOP ( 'NONE', ( #51442, #55438, #12986, #29966 ) ) ;
#14967=DIRECTION ( 'NONE',  ( 0.000000000000000000, -0.5000000000000003331, -0.8660254037844384856 ) ) ;
#15014=FACE_BOUND ( 'NONE', #21812, .T. ) ;
#15022=LINE ( 'NONE', #70437, #53861 ) ;
#15083=CARTESIAN_POINT ( 'NONE',  ( 8.321939743097969355, 92.04720212734648044, 118.0645406551164029 ) ) ;
#15125=CARTESIAN_POINT ( 'NONE',  ( -492.0614999999999668, 93.66249999999999432, 90.48749999999999716 ) ) ;
#15137=CIRCLE ( 'NONE', #26724, 16.33514202138210791 ) ;
#15161=DIRECTION ( 'NONE',  ( 0.000000000000000000, 0.000000000000000000, 1.000000000000000000 ) ) ;
#15162=ORIENTED_EDGE ( 'NONE', *, *, #19149, .F. ) ;
#15195=CARTESIAN_POINT ( 'NONE',  ( -48.02966122971776741, 353.0471713899363522, 75.53254848357481421 ) ) ;
#15286=ORIENTED_EDGE ( 'NONE', *, *, #23094, .T. ) ;
#15300=VERTEX_POINT ( 'NONE', #8613 ) ;
#15319=CARTESIAN_POINT ( 'NONE',  ( 0.000000000000000000, 65.60000000000000853, 0.000000000000000000 ) ) ;
#15326=LINE ( 'NONE', #9398, #23517 ) ;
#15333=AXIS2_PLACEMENT_3D ( 'NONE', #7732, #89514, #62689 ) ;
#15348=LINE ( 'NONE', #35314, #83019 ) ;
#15378=VERTEX_POINT ( 'NONE', #5362 ) ;
#15386=ORIENTED_EDGE ( 'NONE', *, *, #86162, .F. ) ;
#15407=SURFACE_STYLE_FILL_AREA ( #15846 ) ;
#15428=ORIENTED_EDGE ( 'NONE', *, *, #78336, .T. ) ;
#15444=ORIENTED_EDGE ( 'NONE', *, *, #84282, .F. ) ;
#15456=DIRECTION ( 'NONE',  ( -1.000000000000000000, 0.000000000000000000, 0.000000000000000000 ) ) ;
#15463=CARTESIAN_POINT ( 'NONE',  ( 12.70000000000000107, 81.71003749631398705, 117.8738102209307925 ) ) ;
#15499=CARTESIAN_POINT ( 'NONE',  ( -9.487324347909602551, 74.21786271237625954, 117.9765759210854554 ) ) ;
#15525=EDGE_CURVE ( 'NONE', #23402, #22043, #35744, .T. ) ;
#15530=AXIS2_PLACEMENT_3D ( 'NONE', #10819, #53010, #80779 ) ;
#15536=DIRECTION ( 'NONE',  ( -1.000000000000000000, 0.000000000000000000, 0.000000000000000000 ) ) ;
#15585=DIRECTION ( 'NONE',  ( 0.000000000000000000, 1.000000000000000000, -2.731847993664264698E-16 ) ) ;
#15590=ORIENTED_EDGE ( 'NONE', *, *, #49985, .F. ) ;
#15662=VERTEX_POINT ( 'NONE', #46113 ) ;
#15672=ORIENTED_EDGE ( 'NONE', *, *, #53197, .T. ) ;
#15695=ORIENTED_EDGE ( 'NONE', *, *, #20376, .F. ) ;
#15715=DIRECTION ( 'NONE',  ( 0.000000000000000000, 0.000000000000000000, -1.000000000000000000 ) ) ;
#15746=EDGE_CURVE ( 'NONE', #12182, #58138, #18881, .T. ) ;
#15767=ORIENTED_EDGE ( 'NONE', *, *, #74202, .F. ) ;
#15807=LINE ( 'NONE', #50759, #598 ) ;
#15812=CARTESIAN_POINT ( 'NONE',  ( -544.5124999999999318, 53.97500000000000142, 50.79999999999999716 ) ) ;
#15820=ORIENTED_EDGE ( 'NONE', *, *, #71493, .F. ) ;
#15842=ORIENTED_EDGE ( 'NONE', *, *, #59501, .T. ) ;
#15846=FILL_AREA_STYLE ('',( #57153 ) ) ;
#15857=CARTESIAN_POINT ( 'NONE',  ( -487.2989999999999782, 21.43125000000029701, 15.23694598552314972 ) ) ;
#15860=AXIS2_PLACEMENT_3D ( 'NONE', #52845, #79286, #85656 ) ;
#15878=EDGE_CURVE ( 'NONE', #84869, #1472, #88834, .T. ) ;
#15924=ORIENTED_EDGE ( 'NONE', *, *, #22345, .F. ) ;
#15931=ORIENTED_EDGE ( 'NONE', *, *, #23588, .T. ) ;
#15948=LINE ( 'NONE', #44968, #22470 ) ;
#15963=CARTESIAN_POINT ( 'NONE',  ( 70.63919639214310564, 91.07499999999996021, 53.63573739454427880 ) ) ;
#16011=DIRECTION ( 'NONE',  ( -0.000000000000000000, 1.000000000000000000, -0.000000000000000000 ) ) ;
#16017=VERTEX_POINT ( 'NONE', #86375 ) ;
#16029=DIRECTION ( 'NONE',  ( -1.000000000000000000, 0.000000000000000000, 0.000000000000000000 ) ) ;
#16030=CARTESIAN_POINT ( 'NONE',  ( -215.9000000000000057, 3.174999999999999822, 142.8750000000000000 ) ) ;
#16059=PLANE ( 'NONE',  #50876 ) ;
#16070=CARTESIAN_POINT ( 'NONE',  ( -254.0000000000000000, 104.7749999999999915, 142.8750000000000000 ) ) ;
#16092=LINE ( 'NONE', #56044, #77921 ) ;
#16128=ORIENTED_EDGE ( 'NONE', *, *, #10848, .T. ) ;
#16133=VECTOR ( 'NONE', #6881, 1000.000000000000000 ) ;
#16174=ORIENTED_EDGE ( 'NONE', *, *, #38639, .T. ) ;
#16194=VERTEX_POINT ( 'NONE', #33189 ) ;
#16198=DIRECTION ( 'NONE',  ( -0.000000000000000000, 1.000000000000000000, -0.000000000000000000 ) ) ;
#16242=VERTEX_POINT ( 'NONE', #45446 ) ;
#16243=DIRECTION ( 'NONE',  ( -0.000000000000000000, -1.000000000000000000, -0.000000000000000000 ) ) ;
#16259=DIRECTION ( 'NONE',  ( 0.000000000000000000, 0.000000000000000000, 1.000000000000000000 ) ) ;
#16305=DIRECTION ( 'NONE',  ( 0.000000000000000000, 6.982966722218760189E-15, -1.000000000000000000 ) ) ;
#16313=ORIENTED_EDGE ( 'NONE', *, *, #22132, .T. ) ;
#16323=CARTESIAN_POINT ( 'NONE',  ( 4.665904304751416087E-15, 65.60000000000000853, -38.10000000000000142 ) ) ;
#16367=DIRECTION ( 'NONE',  ( 1.000000000000000000, 0.000000000000000000, 0.000000000000000000 ) ) ;
#16377=DIRECTION ( 'NONE',  ( 1.000000000000000000, 0.000000000000000000, 0.000000000000000000 ) ) ;
#16379=ADVANCED_FACE ( 'NONE', ( #74071 ), #53600, .T. ) ;
#16393=DIRECTION ( 'NONE',  ( 1.000000000000000000, 0.000000000000000000, 0.000000000000000000 ) ) ;
#16428=CARTESIAN_POINT ( 'NONE',  ( 4.081702869980341042, 94.58342596962857840, 118.4863875214337838 ) ) ;
#16522=VECTOR ( 'NONE', #81918, 1000.000000000000114 ) ;
#16524=DIRECTION ( 'NONE',  ( -1.000000000000000000, 7.570719237730541270E-15, 0.000000000000000000 ) ) ;
#16530=DIRECTION ( 'NONE',  ( 0.7071067811865660024, 0.000000000000000000, 0.7071067811865291430 ) ) ;
#16566=ORIENTED_EDGE ( 'NONE', *, *, #68493, .F. ) ;
#16571=AXIS2_PLACEMENT_3D ( 'NONE', #64300, #36137, #83396 ) ;
#16579=DIRECTION ( 'NONE',  ( 0.000000000000000000, 0.000000000000000000, 1.000000000000000000 ) ) ;
#16591=LINE ( 'NONE', #37921, #3529 ) ;
#16615=VECTOR ( 'NONE', #78940, 1000.000000000000000 ) ;
#16628=VERTEX_POINT ( 'NONE', #55283 ) ;
#16639=DIRECTION ( 'NONE',  ( -0.000000000000000000, 1.000000000000000000, -0.000000000000000000 ) ) ;
#16645=ORIENTED_EDGE ( 'NONE', *, *, #34064, .T. ) ;
#16649=EDGE_CURVE ( 'NONE', #56710, #43418, #6269, .T. ) ;
#16657=ORIENTED_EDGE ( 'NONE', *, *, #14935, .F. ) ;
#16690=VECTOR ( 'NONE', #79766, 1000.000000000000000 ) ;
#16703=ORIENTED_EDGE ( 'NONE', *, *, #19132, .F. ) ;
#16707=PLANE ( 'NONE',  #23883 ) ;
#16736=ORIENTED_EDGE ( 'NONE', *, *, #4045, .F. ) ;
#16780=VERTEX_POINT ( 'NONE', #68349 ) ;
#16817=ORIENTED_EDGE ( 'NONE', *, *, #88605, .T. ) ;
#16831=CARTESIAN_POINT ( 'NONE',  ( -446.0240000000000009, 93.66249999999999432, 11.11250000000040217 ) ) ;
#16834=CYLINDRICAL_SURFACE ( 'NONE', #37358, 12.60000000000000142 ) ;
#16841=ORIENTED_EDGE ( 'NONE', *, *, #12576, .T. ) ;
#16868=LINE ( 'NONE', #3244, #22728 ) ;
#16871=CARTESIAN_POINT ( 'NONE',  ( 3.284115064261067030, 94.82510599261892992, 118.5111763271416692 ) ) ;
#16884=AXIS2_PLACEMENT_3D ( 'NONE', #47954, #74791, #33897 ) ;
#16899=DIRECTION ( 'NONE',  ( -1.000000000000000000, 0.000000000000000000, 0.000000000000000000 ) ) ;
#16953=VERTEX_POINT ( 'NONE', #1096 ) ;
#16962=AXIS2_PLACEMENT_3D ( 'NONE', #18680, #67270, #46359 ) ;
#16986=CARTESIAN_POINT ( 'NONE',  ( -492.0614999999999668, 93.66249999999999432, 90.48749999999999716 ) ) ;
#17036=DIRECTION ( 'NONE',  ( 0.000000000000000000, -1.682382052829014912E-15, -1.000000000000000000 ) ) ;
#17075=ORIENTED_EDGE ( 'NONE', *, *, #73566, .T. ) ;
#17093=EDGE_CURVE ( 'NONE', #16780, #72546, #17223, .T. ) ;
#17096=VECTOR ( 'NONE', #69144, 1000.000000000000000 ) ;
#17103=DIRECTION ( 'NONE',  ( 1.000000000000000000, 0.000000000000000000, 0.000000000000000000 ) ) ;
#17109=EDGE_CURVE ( 'NONE', #274, #45431, #89008, .T. ) ;
#17134=DIRECTION ( 'NONE',  ( 0.000000000000000000, 1.000000000000000000, 0.000000000000000000 ) ) ;
#17187=CARTESIAN_POINT ( 'NONE',  ( -469.3583484187089994, 53.97500000000000142, 3.174999999999999822 ) ) ;
#17223=LINE ( 'NONE', #79460, #17936 ) ;
#17269=CARTESIAN_POINT ( 'NONE',  ( -12.60000000000000142, 82.54999999999999716, 92.46299999999996544 ) ) ;
#17272=ORIENTED_EDGE ( 'NONE', *, *, #83532, .F. ) ;
#17292=DIRECTION ( 'NONE',  ( 0.2884130866282238470, 0.7071067811865494601, -0.6456143519637539407 ) ) ;
#17342=PLANE ( 'NONE',  #72519 ) ;
#17377=FACE_OUTER_BOUND ( 'NONE', #65926, .T. ) ;
#17387=AXIS2_PLACEMENT_3D ( 'NONE', #2958, #9773, #37477 ) ;
#17395=CARTESIAN_POINT ( 'NONE',  ( -47.18030668273772221, 93.07500000000001705, 75.34738655934135920 ) ) ;
#17403=EDGE_CURVE ( 'NONE', #74897, #62421, #6331, .T. ) ;
#17419=EDGE_CURVE ( 'NONE', #60827, #83591, #44055, .T. ) ;
#17427=EDGE_CURVE ( 'NONE', #75163, #64560, #53711, .T. ) ;
#17475=DIRECTION ( 'NONE',  ( 0.000000000000000000, 0.000000000000000000, -1.000000000000000000 ) ) ;
#17513=VECTOR ( 'NONE', #11609, 1000.000000000000000 ) ;
#17514=EDGE_CURVE ( 'NONE', #12332, #2162, #81759, .T. ) ;
#17533=ADVANCED_FACE ( 'NONE', ( #21471 ), #562, .F. ) ;
#17547=DIRECTION ( 'NONE',  ( 1.000000000000000000, 0.000000000000000000, 0.000000000000000000 ) ) ;
#17573=ORIENTED_EDGE ( 'NONE', *, *, #9055, .T. ) ;
#17578=FACE_BOUND ( 'NONE', #77234, .T. ) ;
#17632=LINE ( 'NONE', #31695, #21446 ) ;
#17684=AXIS2_PLACEMENT_3D ( 'NONE', #61127, #19356, #47928 ) ;
#17690=CARTESIAN_POINT ( 'NONE',  ( -446.0240000000000009, 104.7749999999999915, -1.387778780781445991E-14 ) ) ;
#17694=DIRECTION ( 'NONE',  ( 0.000000000000000000, -0.4999999999999921174, -0.8660254037844431485 ) ) ;
#17699=LINE ( 'NONE', #45379, #20521 ) ;
#17700=VERTEX_POINT ( 'NONE', #44574 ) ;
#17753=PLANE ( 'NONE',  #19795 ) ;
#17759=CARTESIAN_POINT ( 'NONE',  ( 0.8389232435964502077, 95.25000000000004263, 118.5560000000000542 ) ) ;
#17788=VERTEX_POINT ( 'NONE', #72747 ) ;
#17792=EDGE_CURVE ( 'NONE', #49775, #29846, #3701, .T. ) ;
#17857=LINE ( 'NONE', #23801, #37114 ) ;
#17936=VECTOR ( 'NONE', #72183, 1000.000000000000000 ) ;
#17946=LINE ( 'NONE', #11131, #22966 ) ;
#17959=EDGE_CURVE ( 'NONE', #51171, #14599, #13220, .T. ) ;
#17978=VECTOR ( 'NONE', #73931, 1000.000000000000000 ) ;
#18013=DIRECTION ( 'NONE',  ( -0.9419738712670565617, 0.000000000000000000, -0.3356862014592719157 ) ) ;
#18055=FACE_OUTER_BOUND ( 'NONE', #25861, .T. ) ;
#18099=EDGE_LOOP ( 'NONE', ( #43509, #77113 ) ) ;
#18103=ORIENTED_EDGE ( 'NONE', *, *, #17419, .F. ) ;
#18167=CIRCLE ( 'NONE', #45763, 4.762500000000001066 ) ;
#18177=DIRECTION ( 'NONE',  ( 1.000000000000000000, 0.000000000000000000, 0.000000000000000000 ) ) ;
#18191=DIRECTION ( 'NONE',  ( 0.000000000000000000, 0.000000000000000000, -1.000000000000000000 ) ) ;
#18198=CARTESIAN_POINT ( 'NONE',  ( 12.70000000000000107, 82.54999999999999716, 117.8738102209307641 ) ) ;
#18225=CARTESIAN_POINT ( 'NONE',  ( 70.63919639214310564, 49.07499999999999574, -33.74458626278666884 ) ) ;
#18232=DIRECTION ( 'NONE',  ( 1.000000000000000000, 0.000000000000000000, 0.000000000000000000 ) ) ;
#18243=VERTEX_POINT ( 'NONE', #82158 ) ;
#18246=ORIENTED_EDGE ( 'NONE', *, *, #39821, .T. ) ;
#18305=VERTEX_POINT ( 'NONE', #74875 ) ;
#18362=CARTESIAN_POINT ( 'NONE',  ( -458.3598257906459708, 47.62500000000000000, -3.174999999999999822 ) ) ;
#18426=EDGE_LOOP ( 'NONE', ( #26895, #13101, #15695, #36841 ) ) ;
#18439=AXIS2_PLACEMENT_3D ( 'NONE', #23268, #65463, #51365 ) ;
#18455=ORIENTED_EDGE ( 'NONE', *, *, #12511, .T. ) ;
#18469=CARTESIAN_POINT ( 'NONE',  ( -55.95243198108136085, 55.97500000000000142, 70.69974874213239957 ) ) ;
#18485=ORIENTED_EDGE ( 'NONE', *, *, #26714, .T. ) ;
#18510=EDGE_CURVE ( 'NONE', #60827, #53045, #30307, .T. ) ;
#18514=CARTESIAN_POINT ( 'NONE',  ( -544.5124999999999318, 53.97500000000000142, 50.79999999999999716 ) ) ;
#18528=PLANE ( 'NONE',  #8826 ) ;
#18541=AXIS2_PLACEMENT_3D ( 'NONE', #89081, #69085, #28635 ) ;
#18563=DIRECTION ( 'NONE',  ( 0.000000000000000000, 0.000000000000000000, 1.000000000000000000 ) ) ;
#18572=CARTESIAN_POINT ( 'NONE',  ( -446.0240000000000009, 93.66249999999999432, 15.87500000000039968 ) ) ;
#18618=AXIS2_PLACEMENT_3D ( 'NONE', #18956, #21079, #6551 ) ;
#18646=CARTESIAN_POINT ( 'NONE',  ( 69.97247222095467123, 91.74172417118840883, -53.74920436177191618 ) ) ;
#18652=EDGE_CURVE ( 'NONE', #296, #27915, #45246, .T. ) ;
#18680=CARTESIAN_POINT ( 'NONE',  ( 0.000000000000000000, 92.07499999999998863, 0.000000000000000000 ) ) ;
#18691=CARTESIAN_POINT ( 'NONE',  ( -40.89999999999999858, 53.97500000000000142, 50.79999999999999716 ) ) ;
#18704=ADVANCED_FACE ( 'NONE', ( #32512 ), #12997, .F. ) ;
#18713=FACE_OUTER_BOUND ( 'NONE', #8426, .T. ) ;
#18748=CARTESIAN_POINT ( 'NONE',  ( -240.5296158183964792, 93.66249999999999432, 15.87500000000039968 ) ) ;
#18750=DIRECTION ( 'NONE',  ( -0.000000000000000000, 1.000000000000000000, -0.000000000000000000 ) ) ;
#18761=VECTOR ( 'NONE', #57359, 1000.000000000000000 ) ;
#18768=CARTESIAN_POINT ( 'NONE',  ( -12.17775636522063643, 85.81091203684010793, 117.7279047925309925 ) ) ;
#18771=ORIENTED_EDGE ( 'NONE', *, *, #3742, .T. ) ;
#18780=ORIENTED_EDGE ( 'NONE', *, *, #67114, .F. ) ;
#18802=EDGE_LOOP ( 'NONE', ( #4522, #46646, #64036, #1412 ) ) ;
#18836=DIRECTION ( 'NONE',  ( 0.000000000000000000, 0.000000000000000000, -1.000000000000000000 ) ) ;
#18858=DIRECTION ( 'NONE',  ( 0.000000000000000000, 0.000000000000000000, 1.000000000000000000 ) ) ;
#18861=CARTESIAN_POINT ( 'NONE',  ( -450.8499999999999659, 53.97500000000000142, -1.387778780781445991E-14 ) ) ;
#18868=ORIENTED_EDGE ( 'NONE', *, *, #10614, .F. ) ;
#18876=AXIS2_PLACEMENT_3D ( 'NONE', #3495, #3061, #18013 ) ;
#18878=EDGE_LOOP ( 'NONE', ( #44458, #7500, #66585 ) ) ;
#18881=LINE ( 'NONE', #11162, #29374 ) ;
#18915=LINE ( 'NONE', #69641, #13054 ) ;
#18934=FACE_BOUND ( 'NONE', #58436, .T. ) ;
#18944=DIRECTION ( 'NONE',  ( 0.9586846635221889512, 0.000000000000000000, -0.2844709403917162205 ) ) ;
#18946=LINE ( 'NONE', #6220, #26435 ) ;
#18956=CARTESIAN_POINT ( 'NONE',  ( -487.2989999999999782, 14.28750000000036025, 2.863608028952925100 ) ) ;
#18983=EDGE_CURVE ( 'NONE', #18305, #70548, #81507, .T. ) ;
#18985=APPLICATION_CONTEXT ( 'automotive_design' ) ;
#18987=ORIENTED_EDGE ( 'NONE', *, *, #40043, .F. ) ;
#19008=VECTOR ( 'NONE', #28056, 1000.000000000000000 ) ;
#19020=CYLINDRICAL_SURFACE ( 'NONE', #57671, 118.3560000000000088 ) ;
#19034=DIRECTION ( 'NONE',  ( 0.3356862014592719712, 0.000000000000000000, -0.9419738712670565617 ) ) ;
#19061=CARTESIAN_POINT ( 'NONE',  ( -47.18030668273772221, 100.5999999999999659, 75.34738655934135920 ) ) ;
#19077=EDGE_LOOP ( 'NONE', ( #2687, #27498, #81556, #75523 ) ) ;
#19110=CARTESIAN_POINT ( 'NONE',  ( -446.0240000000000009, 53.97500000000000142, 50.79999999999999716 ) ) ;
#19115=EDGE_CURVE ( 'NONE', #87454, #71894, #30645, .T. ) ;
#19128=ORIENTED_EDGE ( 'NONE', *, *, #78023, .T. ) ;
#19132=EDGE_CURVE ( 'NONE', #15662, #10687, #75455, .T. ) ;
#19133=AXIS2_PLACEMENT_3D ( 'NONE', #79462, #72185, #24485 ) ;
#19149=EDGE_CURVE ( 'NONE', #50592, #74753, #21383, .T. ) ;
#19150=ORIENTED_EDGE ( 'NONE', *, *, #7988, .F. ) ;
#19163=PLANE ( 'NONE',  #68949 ) ;
#19179=DIRECTION ( 'NONE',  ( 1.000000000000000000, 0.000000000000000000, 0.000000000000000000 ) ) ;
#19184=CARTESIAN_POINT ( 'NONE',  ( -479.3614999999999782, 97.78694598552370110, 18.25625000000050235 ) ) ;
#19196=EDGE_LOOP ( 'NONE', ( #83103, #4620, #74826, #20047 ) ) ;
#19218=ORIENTED_EDGE ( 'NONE', *, *, #48741, .T. ) ;
#19260=DIRECTION ( 'NONE',  ( 0.000000000000000000, 0.000000000000000000, -1.000000000000000000 ) ) ;
#19265=DIRECTION ( 'NONE',  ( 0.000000000000000000, 0.000000000000000000, 1.000000000000000000 ) ) ;
#19286=DIRECTION ( 'NONE',  ( 0.7071067811865561215, -0.000000000000000000, -0.7071067811865389130 ) ) ;
#19331=ORIENTED_EDGE ( 'NONE', *, *, #77723, .T. ) ;
#19356=DIRECTION ( 'NONE',  ( -0.000000000000000000, 1.000000000000000000, 0.000000000000000000 ) ) ;
#19368=DIRECTION ( 'NONE',  ( -1.000000000000000000, 0.000000000000000000, 0.000000000000000000 ) ) ;
#19404=CARTESIAN_POINT ( 'NONE',  ( -487.2989999999999782, 85.41360802895360393, 11.11250000000036131 ) ) ;
#19430=VERTEX_POINT ( 'NONE', #17690 ) ;
#19452=ORIENTED_EDGE ( 'NONE', *, *, #48032, .T. ) ;
#19470=DIRECTION ( 'NONE',  ( 0.000000000000000000, -1.000000000000000000, 0.000000000000000000 ) ) ;
#19472=DIRECTION ( 'NONE',  ( 0.000000000000000000, 0.000000000000000000, -1.000000000000000000 ) ) ;
#19491=FACE_OUTER_BOUND ( 'NONE', #29064, .T. ) ;
#19524=VERTEX_POINT ( 'NONE', #53055 ) ;
#19537=DIRECTION ( 'NONE',  ( -0.000000000000000000, 1.000000000000000000, -0.000000000000000000 ) ) ;
#19540=EDGE_LOOP ( 'NONE', ( #74056, #14055, #89349, #13941 ) ) ;
#19550=DIRECTION ( 'NONE',  ( 1.000000000000000000, 0.000000000000000000, 0.000000000000000000 ) ) ;
#19566=CARTESIAN_POINT ( 'NONE',  ( -487.2989999999999782, 6.038608028953049711, 90.48749999999999716 ) ) ;
#19571=VERTEX_POINT ( 'NONE', #11312 ) ;
#19574=EDGE_LOOP ( 'NONE', ( #24145, #63521, #45305 ) ) ;
#19584=VERTEX_POINT ( 'NONE', #39013 ) ;
#19590=DIRECTION ( 'NONE',  ( -0.2884130866282236250, -0.7071067811865507924, 0.6456143519637524975 ) ) ;
#19613=CARTESIAN_POINT ( 'NONE',  ( -451.6120000000000232, 53.97500000000000142, -3.174999999999999822 ) ) ;
#19615=DIRECTION ( 'NONE',  ( 0.000000000000000000, 6.920681583949466031E-15, -1.000000000000000000 ) ) ;
#19619=CARTESIAN_POINT ( 'NONE',  ( -487.2989999999999782, 93.66249999999999432, 15.87500000000039968 ) ) ;
#19646=DIRECTION ( 'NONE',  ( 0.000000000000000000, 0.000000000000000000, 1.000000000000000000 ) ) ;
#19651=EDGE_CURVE ( 'NONE', #79764, #36007, #25120, .T. ) ;
#19663=CIRCLE ( 'NONE', #79147, 88.90000000000000568 ) ;
#19669=CARTESIAN_POINT ( 'NONE',  ( -492.0614999999999668, 14.28749999999982201, 90.48749999999999716 ) ) ;
#19707=CARTESIAN_POINT ( 'NONE',  ( -487.2989999999999782, 7.143750000000339995, 6.988054014476278830 ) ) ;
#19739=ORIENTED_EDGE ( 'NONE', *, *, #58084, .T. ) ;
#19778=DIRECTION ( 'NONE',  ( 0.000000000000000000, -0.8660254037844351549, -0.5000000000000061062 ) ) ;
#19785=EDGE_CURVE ( 'NONE', #1301, #51309, #37586, .T. ) ;
#19792=VECTOR ( 'NONE', #24854, 1000.000000000000000 ) ;
#19795=AXIS2_PLACEMENT_3D ( 'NONE', #73150, #78218, #38631 ) ;
#19806=DIRECTION ( 'NONE',  ( 0.000000000000000000, 0.000000000000000000, 1.000000000000000000 ) ) ;
#19810=VERTEX_POINT ( 'NONE', #1729 ) ;
#19821=DIRECTION ( 'NONE',  ( 0.000000000000000000, 0.000000000000000000, -1.000000000000000000 ) ) ;
#19829=DIRECTION ( 'NONE',  ( 1.000000000000000000, 0.000000000000000000, 0.000000000000000000 ) ) ;
#19838=LINE ( 'NONE', #54772, #44862 ) ;
#19840=CARTESIAN_POINT ( 'NONE',  ( -48.02966122971776741, 100.5999999999999659, 75.53254848357481421 ) ) ;
#19841=DIRECTION ( 'NONE',  ( 1.000000000000000000, 0.000000000000000000, 0.000000000000000000 ) ) ;
#19876=DIRECTION ( 'NONE',  ( -0.000000000000000000, -0.000000000000000000, 1.000000000000000000 ) ) ;
#19885=EDGE_LOOP ( 'NONE', ( #43858, #53294 ) ) ;
#19892=FACE_BOUND ( 'NONE', #54899, .T. ) ;
#19933=ORIENTED_EDGE ( 'NONE', *, *, #70421, .F. ) ;
#19934=LINE ( 'NONE', #33991, #65563 ) ;
#19940=CIRCLE ( 'NONE', #85263, 11.17600000000001970 ) ;
#19943=ORIENTED_EDGE ( 'NONE', *, *, #38767, .F. ) ;
#19953=EDGE_CURVE ( 'NONE', #2949, #36750, #58893, .T. ) ;
#20011=CARTESIAN_POINT ( 'NONE',  ( -31.27367473141074683, 54.97499999999995879, 74.45358409497265484 ) ) ;
#20047=ORIENTED_EDGE ( 'NONE', *, *, #85745, .T. ) ;
#20062=CARTESIAN_POINT ( 'NONE',  ( -4.049533659350667669, 70.61131560177412325, 118.2873649127880071 ) ) ;
#20076=AXIS2_PLACEMENT_3D ( 'NONE', #68539, #34000, #7210 ) ;
#20093=DIRECTION ( 'NONE',  ( -0.000000000000000000, 1.000000000000000000, -0.000000000000000000 ) ) ;
#20116=CARTESIAN_POINT ( 'NONE',  ( -47.02966122971776031, 65.60000000000000853, 108.8289304395572401 ) ) ;
#20122=CARTESIAN_POINT ( 'NONE',  ( -11.79654564977231779, 86.99658319087748737, 117.7667590573388026 ) ) ;
#20127=CARTESIAN_POINT ( 'NONE',  ( 0.000000000000000000, 101.5999999999999943, 0.000000000000000000 ) ) ;
#20178=VECTOR ( 'NONE', #48729, 1000.000000000000114 ) ;
#20198=DIRECTION ( 'NONE',  ( 0.000000000000000000, 0.000000000000000000, -1.000000000000000000 ) ) ;
#20203=DIRECTION ( 'NONE',  ( -0.4634479843259246556, -0.000000000000000000, -0.8861241255175470455 ) ) ;
#20206=EDGE_CURVE ( 'NONE', #83591, #36007, #42036, .T. ) ;
#20237=DIRECTION ( 'NONE',  ( 0.000000000000000000, 0.000000000000000000, -1.000000000000000000 ) ) ;
#20302=LINE ( 'NONE', #47971, #53886 ) ;
#20308=EDGE_CURVE ( 'NONE', #53776, #19, #36134, .T. ) ;
#20312=CARTESIAN_POINT ( 'NONE',  ( -487.2989999999999782, 7.143750000000280487, 15.23694598552305024 ) ) ;
#20371=AXIS2_PLACEMENT_3D ( 'NONE', #76375, #56361, #41828 ) ;
#20376=EDGE_CURVE ( 'NONE', #15300, #71038, #3401, .T. ) ;
#20377=FACE_OUTER_BOUND ( 'NONE', #49900, .T. ) ;
#20390=CARTESIAN_POINT ( 'NONE',  ( 6.162975822039154730E-30, 95.25000000000000000, 118.5560000000000116 ) ) ;
#20393=DIRECTION ( 'NONE',  ( 0.000000000000000000, 0.000000000000000000, -1.000000000000000000 ) ) ;
#20395=FACE_OUTER_BOUND ( 'NONE', #6015, .T. ) ;
#20405=FACE_OUTER_BOUND ( 'NONE', #21941, .T. ) ;
#20467=ADVANCED_FACE ( 'NONE', ( #38799 ), #66960, .T. ) ;
#20521=VECTOR ( 'NONE', #44939, 1000.000000000000000 ) ;
#20523=DIRECTION ( 'NONE',  ( -1.000000000000000000, 0.000000000000000000, 0.000000000000000000 ) ) ;
#20547=EDGE_LOOP ( 'NONE', ( #9259, #39798 ) ) ;
#20555=FACE_OUTER_BOUND ( 'NONE', #28795, .T. ) ;
#20558=CYLINDRICAL_SURFACE ( 'NONE', #29982, 3.700000000000001954 ) ;
#20587=ORIENTED_EDGE ( 'NONE', *, *, #19115, .F. ) ;
#20615=CARTESIAN_POINT ( 'NONE',  ( -48.02966122971777452, 66.60000000000003695, 106.4272185163641780 ) ) ;
#20621=CARTESIAN_POINT ( 'NONE',  ( -479.3614999999999782, 18.41194598552320016, 97.63125000000000853 ) ) ;
#20628=DIRECTION ( 'NONE',  ( 1.000000000000000000, 0.000000000000000000, 0.000000000000000000 ) ) ;
#20642=LINE ( 'NONE', #42842, #67465 ) ;
#20655=ADVANCED_FACE ( 'NONE', ( #74670, #22405 ), #36022, .T. ) ;
#20656=DIRECTION ( 'NONE',  ( 0.000000000000000000, 0.000000000000000000, -1.000000000000000000 ) ) ;
#20684=VECTOR ( 'NONE', #77424, 1000.000000000000000 ) ;
#20690=ORIENTED_EDGE ( 'NONE', *, *, #76279, .F. ) ;
#20692=CARTESIAN_POINT ( 'NONE',  ( 70.63919639214310564, 93.07500000000001705, 56.85413200336923012 ) ) ;
#20716=LINE ( 'NONE', #88871, #12857 ) ;
#20766=FACE_OUTER_BOUND ( 'NONE', #24540, .T. ) ;
#20775=EDGE_CURVE ( 'NONE', #78144, #75163, #36355, .T. ) ;
#20777=ADVANCED_FACE ( 'NONE', ( #6367 ), #34058, .F. ) ;
#20808=EDGE_CURVE ( 'NONE', #10687, #76744, #1357, .T. ) ;
#20844=VECTOR ( 'NONE', #30358, 1000.000000000000227 ) ;
#20847=CIRCLE ( 'NONE', #71629, 16.33514202138213633 ) ;
#20858=AXIS2_PLACEMENT_3D ( 'NONE', #67592, #41210, #74861 ) ;
#20876=FACE_OUTER_BOUND ( 'NONE', #57860, .T. ) ;
#20897=CARTESIAN_POINT ( 'NONE',  ( -46.60773131249376178, 91.07499999999996021, -44.42500552774628630 ) ) ;
#20951=CARTESIAN_POINT ( 'NONE',  ( -479.3614999999999782, 100.8062500000000057, 94.61194598552329182 ) ) ;
#20961=DIRECTION ( 'NONE',  ( 0.000000000000000000, -0.8660254037844382635, -0.5000000000000008882 ) ) ;
#20964=VECTOR ( 'NONE', #54038, 1000.000000000000000 ) ;
#20995=CARTESIAN_POINT ( 'NONE',  ( -24.20305689751608824, 53.97499999999997300, 58.62596543806478877 ) ) ;
#21014=CARTESIAN_POINT ( 'NONE',  ( -254.0000000000000000, 14.28749999999982201, 95.25000000000000000 ) ) ;
#21062=CARTESIAN_POINT ( 'NONE',  ( -64.50026246089650783, 148.4450814996825443, 59.61038444174924678 ) ) ;
#21079=DIRECTION ( 'NONE',  ( -0.000000000000000000, 0.4999999999999985567, 0.8660254037844394848 ) ) ;
#21115=EDGE_LOOP ( 'NONE', ( #12510, #9408, #70796, #26825 ) ) ;
#21116=VECTOR ( 'NONE', #1314, 1000.000000000000114 ) ;
#21117=CARTESIAN_POINT ( 'NONE',  ( -41.60202597009397607, 65.59999999999998010, 50.85338361873603219 ) ) ;
#21144=VERTEX_POINT ( 'NONE', #86942 ) ;
#21179=PLANE ( 'NONE',  #931 ) ;
#21209=ORIENTED_EDGE ( 'NONE', *, *, #9520, .T. ) ;
#21236=VERTEX_POINT ( 'NONE', #66473 ) ;
#21278=ORIENTED_EDGE ( 'NONE', *, *, #78565, .T. ) ;
#21305=CARTESIAN_POINT ( 'NONE',  ( -1.790903581468949841E-22, 95.14999999999999147, 118.3560000000000088 ) ) ;
#21365=DIRECTION ( 'NONE',  ( -1.000000000000000000, 0.000000000000000000, 0.000000000000000000 ) ) ;
#21369=LINE ( 'NONE', #49044, #11695 ) ;
#21371=CARTESIAN_POINT ( 'NONE',  ( 8.391117282579658720, 72.98104651172248225, 118.2601343779861622 ) ) ;
#21383=LINE ( 'NONE', #26837, #39060 ) ;
#21415=LINE ( 'NONE', #26870, #3737 ) ;
#21440=ADVANCED_FACE ( 'NONE', ( #78254 ), #3273, .F. ) ;
#21443=ORIENTED_EDGE ( 'NONE', *, *, #46594, .T. ) ;
#21446=VECTOR ( 'NONE', #45311, 1000.000000000000000 ) ;
#21471=FACE_OUTER_BOUND ( 'NONE', #74159, .T. ) ;
#21487=ADVANCED_FACE ( 'NONE', ( #70526 ), #1931, .T. ) ;
#21499=DIRECTION ( 'NONE',  ( 0.000000000000000000, 0.000000000000000000, 1.000000000000000000 ) ) ;
#21504=EDGE_CURVE ( 'NONE', #24976, #58319, #81370, .T. ) ;
#21521=DIRECTION ( 'NONE',  ( -0.9130365726098600421, 0.000000000000000000, -0.4078776986755215939 ) ) ;
#21533=DIRECTION ( 'NONE',  ( 1.821299053822143307E-16, 0.000000000000000000, -1.000000000000000000 ) ) ;
#21547=VECTOR ( 'NONE', #44269, 1000.000000000000114 ) ;
#21573=FACE_OUTER_BOUND ( 'NONE', #44057, .T. ) ;
#21583=ORIENTED_EDGE ( 'NONE', *, *, #3017, .F. ) ;
#21584=VECTOR ( 'NONE', #24061, 1000.000000000000000 ) ;
#21687=EDGE_CURVE ( 'NONE', #70548, #18305, #67923, .T. ) ;
#21689=DIRECTION ( 'NONE',  ( -0.000000000000000000, 0.4999999999999995004, 0.8660254037844390407 ) ) ;
#21712=CARTESIAN_POINT ( 'NONE',  ( 0.000000000000000000, 101.6000000000000227, 89.90000000000000568 ) ) ;
#21717=ORIENTED_EDGE ( 'NONE', *, *, #83027, .T. ) ;
#21738=DIRECTION ( 'NONE',  ( 0.000000000000000000, 0.000000000000000000, 1.000000000000000000 ) ) ;
#21761=DIRECTION ( 'NONE',  ( 0.000000000000000000, 0.8660254037844387076, 0.4999999999999998890 ) ) ;
#21772=( NAMED_UNIT ( * ) PLANE_ANGLE_UNIT ( ) SI_UNIT ( $, .RADIAN. ) );
#21780=CARTESIAN_POINT ( 'NONE',  ( -76.55155505517849690, 55.04324208698172782, 30.82815564505935768 ) ) ;
#21812=EDGE_LOOP ( 'NONE', ( #911, #50003 ) ) ;
#21838=DIRECTION ( 'NONE',  ( 1.000000000000000000, 0.000000000000000000, 0.000000000000000000 ) ) ;
#21854=CARTESIAN_POINT ( 'NONE',  ( -492.0614999999999668, 93.66249999999999432, 11.11250000000040217 ) ) ;
#21907=CARTESIAN_POINT ( 'NONE',  ( 9.497923889340652792, 90.87111597850432076, 117.9757597262406819 ) ) ;
#21909=VECTOR ( 'NONE', #54324, 1000.000000000000000 ) ;
#21941=EDGE_LOOP ( 'NONE', ( #71486, #683, #35256, #15428, #55514, #29818, #31418 ) ) ;
#21956=PLANE ( 'NONE',  #29063 ) ;
#21976=CARTESIAN_POINT ( 'NONE',  ( 0.000000000000000000, 100.5999999999999659, 88.90000000000000568 ) ) ;
#21992=ORIENTED_EDGE ( 'NONE', *, *, #69839, .T. ) ;
#22035=EDGE_CURVE ( 'NONE', #8809, #84439, #80981, .T. ) ;
#22043=VERTEX_POINT ( 'NONE', #2276 ) ;
#22067=ORIENTED_EDGE ( 'NONE', *, *, #43533, .F. ) ;
#22072=ORIENTED_EDGE ( 'NONE', *, *, #66482, .T. ) ;
#22080=CARTESIAN_POINT ( 'NONE',  ( -487.2989999999999782, 14.28750000000023945, 19.36139197104649767 ) ) ;
#22088=FACE_OUTER_BOUND ( 'NONE', #44136, .T. ) ;
#22132=EDGE_CURVE ( 'NONE', #24430, #76709, #58552, .T. ) ;
#22150=ORIENTED_EDGE ( 'NONE', *, *, #22035, .T. ) ;
#22186=DIRECTION ( 'NONE',  ( 0.000000000000000000, 0.000000000000000000, -1.000000000000000000 ) ) ;
#22203=EDGE_CURVE ( 'NONE', #65784, #73034, #11304, .T. ) ;
#22281=PLANE ( 'NONE',  #35648 ) ;
#22308=CARTESIAN_POINT ( 'NONE',  ( -10.69948253693739026, 75.88274056138229184, 117.8716134549241872 ) ) ;
#22345=EDGE_CURVE ( 'NONE', #34343, #82548, #47598, .T. ) ;
#22347=VECTOR ( 'NONE', #76168, 1000.000000000000000 ) ;
#22374=VERTEX_POINT ( 'NONE', #82164 ) ;
#22390=ORIENTED_EDGE ( 'NONE', *, *, #61627, .T. ) ;
#22405=FACE_BOUND ( 'NONE', #22913, .T. ) ;
#22407=CARTESIAN_POINT ( 'NONE',  ( -446.0240000000000009, 3.174999999999999822, -1.387778780781445991E-14 ) ) ;
#22414=FACE_OUTER_BOUND ( 'NONE', #18426, .T. ) ;
#22420=EDGE_CURVE ( 'NONE', #50747, #13441, #54850, .T. ) ;
#22425=PLANE ( 'NONE',  #78357 ) ;
#22427=DIRECTION ( 'NONE',  ( 0.2884130866282256789, -0.7071067811865450192, -0.6456143519637580486 ) ) ;
#22446=AXIS2_PLACEMENT_3D ( 'NONE', #16831, #36384, #64088 ) ;
#22470=VECTOR ( 'NONE', #73123, 1000.000000000000000 ) ;
#22484=CARTESIAN_POINT ( 'NONE',  ( 0.000000000000000000, 100.5999999999999659, 0.000000000000000000 ) ) ;
#22523=ADVANCED_FACE ( 'NONE', ( #42131 ), #8989, .F. ) ;
#22527=CYLINDRICAL_SURFACE ( 'NONE', #27450, 4.762500000000000178 ) ;
#22565=DIRECTION ( 'NONE',  ( 1.821299053822143307E-16, 0.000000000000000000, -1.000000000000000000 ) ) ;
#22579=CARTESIAN_POINT ( 'NONE',  ( -54.73705905482161427, 54.20698630476788082, 70.79887152307878750 ) ) ;
#22609=DIRECTION ( 'NONE',  ( -0.000000000000000000, 1.000000000000000000, 0.000000000000000000 ) ) ;
#22622=CIRCLE ( 'NONE', #89347, 10.41399999999997839 ) ;
#22652=ORIENTED_EDGE ( 'NONE', *, *, #34285, .F. ) ;
#22684=AXIS2_PLACEMENT_3D ( 'NONE', #36110, #63825, #1601 ) ;
#22688=VECTOR ( 'NONE', #26548, 1000.000000000000000 ) ;
#22700=ADVANCED_FACE ( 'NONE', ( #89643 ), #87958, .F. ) ;
#22702=DIRECTION ( 'NONE',  ( 0.000000000000000000, 0.000000000000000000, 1.000000000000000000 ) ) ;
#22717=DIRECTION ( 'NONE',  ( -1.000000000000000000, 0.000000000000000000, 0.000000000000000000 ) ) ;
#22723=CARTESIAN_POINT ( 'NONE',  ( 9.549149029459599092, 74.16675814752574070, 118.1711041523992662 ) ) ;
#22724=VECTOR ( 'NONE', #62117, 1000.000000000000000 ) ;
#22728=VECTOR ( 'NONE', #85485, 1000.000000000000000 ) ;
#22790=EDGE_CURVE ( 'NONE', #71894, #40087, #47825, .T. ) ;
#22815=CARTESIAN_POINT ( 'NONE',  ( 12.52017789511383405, 80.90898357847464695, 117.6920314563592314 ) ) ;
#22862=DIRECTION ( 'NONE',  ( -0.000000000000000000, 1.000000000000000000, -0.000000000000000000 ) ) ;
#22913=EDGE_LOOP ( 'NONE', ( #54430, #69988 ) ) ;
#22926=LINE ( 'NONE', #30172, #5404 ) ;
#22935=DIRECTION ( 'NONE',  ( 0.000000000000000000, 0.4999999999999995004, 0.8660254037844390407 ) ) ;
#22938=AXIS2_PLACEMENT_3D ( 'NONE', #37700, #51742, #38134 ) ;
#22939=EDGE_CURVE ( 'NONE', #7001, #73034, #50522, .T. ) ;
#22947=VERTEX_POINT ( 'NONE', #50970 ) ;
#22966=VECTOR ( 'NONE', #32462, 1000.000000000000000 ) ;
#23008=VECTOR ( 'NONE', #41081, 1000.000000000000000 ) ;
#23020=LINE ( 'NONE', #44769, #32429 ) ;
#23034=EDGE_CURVE ( 'NONE', #53581, #14208, #29635, .T. ) ;
#23043=EDGE_LOOP ( 'NONE', ( #11733, #62699, #66985, #38202 ) ) ;
#23046=VECTOR ( 'NONE', #77033, 1000.000000000000000 ) ;
#23074=CARTESIAN_POINT ( 'NONE',  ( -41.60202597009397607, 76.06518036156089124, 50.85338361873603219 ) ) ;
#23094=EDGE_CURVE ( 'NONE', #67327, #2949, #2095, .T. ) ;
#23125=CIRCLE ( 'NONE', #73851, 4.762500000000002842 ) ;
#23163=DIRECTION ( 'NONE',  ( 0.000000000000000000, 0.000000000000000000, -1.000000000000000000 ) ) ;
#23216=LINE ( 'NONE', #57237, #75490 ) ;
#23220=ORIENTED_EDGE ( 'NONE', *, *, #77082, .T. ) ;
#23225=CARTESIAN_POINT ( 'NONE',  ( -8.311122125636458691, 73.07069292649585179, 118.0642676351586573 ) ) ;
#23268=CARTESIAN_POINT ( 'NONE',  ( -254.0000000000000000, 3.174999999999999822, -41.27499999999999858 ) ) ;
#23278=CARTESIAN_POINT ( 'NONE',  ( 12.60000000000000142, 82.54999999999999716, 117.6834004267381744 ) ) ;
#23293=DIRECTION ( 'NONE',  ( 1.776356839400250465E-15, 0.000000000000000000, -1.000000000000000000 ) ) ;
#23308=ORIENTED_EDGE ( 'NONE', *, *, #64663, .T. ) ;
#23343=CARTESIAN_POINT ( 'NONE',  ( -48.02966122971776741, 91.07499999999996021, 74.26049396966043048 ) ) ;
#23359=DIRECTION ( 'NONE',  ( 0.7071067811865451302, 0.7071067811865500152, -0.000000000000000000 ) ) ;
#23362=CARTESIAN_POINT ( 'NONE',  ( -48.02966122971775320, 100.5999999999999659, -8.747637655308301746E-15 ) ) ;
#23366=CARTESIAN_POINT ( 'NONE',  ( -451.6120000000000232, 53.97500000000000142, -3.174999999999999822 ) ) ;
#23402=VERTEX_POINT ( 'NONE', #59012 ) ;
#23442=LINE ( 'NONE', #35696, #27217 ) ;
#23451=ORIENTED_EDGE ( 'NONE', *, *, #82732, .T. ) ;
#23457=LINE ( 'NONE', #64330, #61359 ) ;
#23465=FACE_OUTER_BOUND ( 'NONE', #21115, .T. ) ;
#23471=CARTESIAN_POINT ( 'NONE',  ( -46.60773131249376178, 91.07499999999996021, -44.42500552774628630 ) ) ;
#23486=ORIENTED_EDGE ( 'NONE', *, *, #20308, .T. ) ;
#23492=ADVANCED_FACE ( 'NONE', ( #34896 ), #27193, .F. ) ;
#23511=CARTESIAN_POINT ( 'NONE',  ( 70.63919639214310564, 65.60000000000000853, 0.000000000000000000 ) ) ;
#23517=VECTOR ( 'NONE', #9849, 1000.000000000000000 ) ;
#23520=CARTESIAN_POINT ( 'NONE',  ( 0.000000000000000000, 49.07499999999999574, 0.000000000000000000 ) ) ;
#23536=CARTESIAN_POINT ( 'NONE',  ( 70.63919639214310564, 49.07499999999999574, -53.97512327982435210 ) ) ;
#23553=DIRECTION ( 'NONE',  ( -0.000000000000000000, -0.000000000000000000, 1.000000000000000000 ) ) ;
#23562=CARTESIAN_POINT ( 'NONE',  ( -254.0000000000000000, 104.7749999999999915, -41.27499999999999858 ) ) ;
#23565=ADVANCED_FACE ( 'NONE', ( #20395 ), #62157, .F. ) ;
#23584=CARTESIAN_POINT ( 'NONE',  ( -54.12775174896490427, 53.97500000000000142, 69.87310403134814862 ) ) ;
#23588=EDGE_CURVE ( 'NONE', #71038, #43418, #56215, .T. ) ;
#23605=ORIENTED_EDGE ( 'NONE', *, *, #33901, .T. ) ;
#23632=LINE ( 'NONE', #77246, #47574 ) ;
#23656=CARTESIAN_POINT ( 'NONE',  ( -11.30280630903569872, 76.96642768152659642, 117.8152258610045351 ) ) ;
#23664=ADVANCED_FACE ( 'NONE', ( #56680 ), #16707, .T. ) ;
#23694=CARTESIAN_POINT ( 'NONE',  ( 0.000000000000000000, 65.60000000000000853, 118.5560000000000116 ) ) ;
#23710=DIRECTION ( 'NONE',  ( 0.000000000000000000, 0.5000000000000007772, -0.8660254037844381525 ) ) ;
#23733=CARTESIAN_POINT ( 'NONE',  ( -47.02966122971775320, 101.5999999999999943, -8.565507749926087908E-15 ) ) ;
#23801=CARTESIAN_POINT ( 'NONE',  ( -487.2989999999999782, 93.66249999999999432, 82.23860802895320887 ) ) ;
#23856=LINE ( 'NONE', #59680, #56397 ) ;
#23883=AXIS2_PLACEMENT_3D ( 'NONE', #23536, #71676, #43490 ) ;
#23901=STYLED_ITEM ( 'NONE', ( #69914 ), #47652 ) ;
#23904=VECTOR ( 'NONE', #157, 1000.000000000000000 ) ;
#23907=CARTESIAN_POINT ( 'NONE',  ( 0.000000000000000000, 65.60000000000000853, 0.000000000000000000 ) ) ;
#23908=VECTOR ( 'NONE', #22862, 1000.000000000000000 ) ;
#23913=ORIENTED_EDGE ( 'NONE', *, *, #2403, .T. ) ;
#23928=PLANE ( 'NONE',  #88804 ) ;
#23946=ORIENTED_EDGE ( 'NONE', *, *, #44070, .T. ) ;
#23988=ORIENTED_EDGE ( 'NONE', *, *, #64438, .F. ) ;
#24011=FACE_OUTER_BOUND ( 'NONE', #60229, .T. ) ;
#24039=VECTOR ( 'NONE', #24554, 1000.000000000000000 ) ;
#24061=DIRECTION ( 'NONE',  ( 1.000000000000000000, 0.000000000000000000, 0.000000000000000000 ) ) ;
#24086=PLANE ( 'NONE',  #42199 ) ;
#24144=CARTESIAN_POINT ( 'NONE',  ( -487.2989999999999782, 18.41194598552320016, 97.63125000000000853 ) ) ;
#24145=ORIENTED_EDGE ( 'NONE', *, *, #6288, .F. ) ;
#24170=ORIENTED_EDGE ( 'NONE', *, *, #27227, .T. ) ;
#24194=DIRECTION ( 'NONE',  ( 0.000000000000000000, -1.000000000000000000, 0.000000000000000000 ) ) ;
#24211=VERTEX_POINT ( 'NONE', #51098 ) ;
#24251=ADVANCED_FACE ( 'NONE', ( #22088 ), #71574, .T. ) ;
#24278=EDGE_CURVE ( 'NONE', #87961, #74649, #4303, .T. ) ;
#24282=CARTESIAN_POINT ( 'NONE',  ( 0.000000000000000000, 65.60000000000000853, 0.000000000000000000 ) ) ;
#24320=PLANE ( 'NONE',  #71689 ) ;
#24336=ORIENTED_EDGE ( 'NONE', *, *, #6244, .T. ) ;
#24343=DIRECTION ( 'NONE',  ( 0.000000000000000000, 0.000000000000000000, 1.000000000000000000 ) ) ;
#24347=AXIS2_PLACEMENT_3D ( 'NONE', #33939, #19876, #27136 ) ;
#24408=CARTESIAN_POINT ( 'NONE',  ( -446.0240000000000009, 3.174999999999999822, -1.387778780781445991E-14 ) ) ;
#24430=VERTEX_POINT ( 'NONE', #68767 ) ;
#24456=VECTOR ( 'NONE', #75685, 1000.000000000000000 ) ;
#24464=LINE ( 'NONE', #52129, #73684 ) ;
#24485=DIRECTION ( 'NONE',  ( 1.000000000000000000, 0.000000000000000000, 0.000000000000000000 ) ) ;
#24490=ORIENTED_EDGE ( 'NONE', *, *, #15878, .F. ) ;
#24502=CIRCLE ( 'NONE', #28849, 38.10000000000000142 ) ;
#24540=EDGE_LOOP ( 'NONE', ( #32078, #55103, #31639, #24955 ) ) ;
#24547=CARTESIAN_POINT ( 'NONE',  ( -41.60202597009397607, 40.59999999999997300, 50.85338361873603219 ) ) ;
#24554=DIRECTION ( 'NONE',  ( 0.000000000000000000, -1.000000000000000000, 0.000000000000000000 ) ) ;
#24579=DIRECTION ( 'NONE',  ( 0.000000000000000000, -0.8660254037844394848, 0.4999999999999986122 ) ) ;
#24586=EDGE_LOOP ( 'NONE', ( #79919, #6358, #33717, #49289 ) ) ;
#24603=VERTEX_POINT ( 'NONE', #14703 ) ;
#24631=VECTOR ( 'NONE', #67332, 1000.000000000000000 ) ;
#24634=DIRECTION ( 'NONE',  ( 0.000000000000000000, 0.000000000000000000, 1.000000000000000000 ) ) ;
#24635=CIRCLE ( 'NONE', #42001, 4.762500000000000178 ) ;
#24644=EDGE_LOOP ( 'NONE', ( #14900, #5671, #63267, #88253, #77028, #54851 ) ) ;
#24649=ADVANCED_FACE ( 'NONE', ( #22414 ), #28776, .F. ) ;
#24658=ADVANCED_FACE ( 'NONE', ( #76470 ), #71015, .F. ) ;
#24671=CARTESIAN_POINT ( 'NONE',  ( 0.000000000000000000, 92.07499999999998863, 0.000000000000000000 ) ) ;
#24691=ORIENTED_EDGE ( 'NONE', *, *, #63650, .F. ) ;
#24725=STYLED_ITEM ( 'NONE', ( #81954 ), #88996 ) ;
#24754=CARTESIAN_POINT ( 'NONE',  ( -41.60202597009397607, 40.59999999999997300, 47.03909206933071374 ) ) ;
#24772=CARTESIAN_POINT ( 'NONE',  ( -479.3614999999999782, 14.28750000000023945, 19.36139197104649767 ) ) ;
#24780=CARTESIAN_POINT ( 'NONE',  ( -47.18030668273772221, 353.0471713899363522, 75.34738655934134499 ) ) ;
#24806=EDGE_LOOP ( 'NONE', ( #74988, #31364, #75986, #43870 ) ) ;
#24819=EDGE_LOOP ( 'NONE', ( #7146, #84746, #78898, #76110 ) ) ;
#24840=DIRECTION ( 'NONE',  ( 0.000000000000000000, 0.000000000000000000, 1.000000000000000000 ) ) ;
#24842=DIRECTION ( 'NONE',  ( 0.000000000000000000, 0.000000000000000000, -1.000000000000000000 ) ) ;
#24854=DIRECTION ( 'NONE',  ( 0.000000000000000000, 1.000000000000000000, 0.000000000000000000 ) ) ;
#24896=DIRECTION ( 'NONE',  ( 0.000000000000000000, 0.000000000000000000, 1.000000000000000000 ) ) ;
#24902=ORIENTED_EDGE ( 'NONE', *, *, #17427, .T. ) ;
#24955=ORIENTED_EDGE ( 'NONE', *, *, #12669, .T. ) ;
#24971=AXIS2_PLACEMENT_3D ( 'NONE', #23074, #16243, #79816 ) ;
#24976=VERTEX_POINT ( 'NONE', #58428 ) ;
#25021=AXIS2_PLACEMENT_3D ( 'NONE', #68375, #89269, #27035 ) ;
#25087=AXIS2_PLACEMENT_3D ( 'NONE', #66828, #74098, #72759 ) ;
#25088=ORIENTED_EDGE ( 'NONE', *, *, #86511, .F. ) ;
#25093=EDGE_CURVE ( 'NONE', #27515, #36325, #5260, .T. ) ;
#25114=LINE ( 'NONE', #48105, #30729 ) ;
#25116=CARTESIAN_POINT ( 'NONE',  ( -9.573302534615132586, 74.16284337107215663, 118.1703442874588319 ) ) ;
#25118=CARTESIAN_POINT ( 'NONE',  ( -487.2989999999999782, 14.28749999999982201, 90.48749999999999716 ) ) ;
#25119=CARTESIAN_POINT ( 'NONE',  ( -544.5124999999999318, 53.97500000000000142, 50.79999999999999716 ) ) ;
#25120=B_SPLINE_CURVE_WITH_KNOTS ( 'NONE', 3,
 ( #40358, #83066, #7195, #13554, #26725, #62594, #83496, #61686, #62145, #89421 ),
 .UNSPECIFIED., .F., .F.,
 ( 4, 3, 3, 4 ),
 ( 0.000000000000000000, 0.0009419788482794725975, 0.001910370295165490350, 0.002878829377803309320 ),
 .UNSPECIFIED. ) ;
#25130=CARTESIAN_POINT ( 'NONE',  ( -4.829308837915109898, 94.20942664101627884, 118.2592588614345885 ) ) ;
#25195=AXIS2_PLACEMENT_3D ( 'NONE', #89620, #62785, #14203 ) ;
#25216=VECTOR ( 'NONE', #71014, 1000.000000000000000 ) ;
#25223=FACE_OUTER_BOUND ( 'NONE', #61595, .T. ) ;
#25262=CARTESIAN_POINT ( 'NONE',  ( -479.3614999999999782, 3.174999999999999822, -1.387778780781445991E-14 ) ) ;
#25264=DIRECTION ( 'NONE',  ( -0.5184798493102225070, -0.5184798493102369399, -0.6799685961266761502 ) ) ;
#25265=EDGE_CURVE ( 'NONE', #970, #77829, #31966, .T. ) ;
#25284=CARTESIAN_POINT ( 'NONE',  ( 0.000000000000000000, 65.60000000000000853, 118.3560000000000088 ) ) ;
#25301=DIRECTION ( 'NONE',  ( 0.4634479843259247112, 0.000000000000000000, 0.8861241255175470455 ) ) ;
#25318=DIRECTION ( 'NONE',  ( 0.000000000000000000, 0.000000000000000000, 1.000000000000000000 ) ) ;
#25354=CARTESIAN_POINT ( 'NONE',  ( -487.2989999999999782, 14.28750000000036025, 2.863608028952925100 ) ) ;
#25360=CIRCLE ( 'NONE', #9485, 3.700000000000001954 ) ;
#25370=EDGE_LOOP ( 'NONE', ( #1487, #3433 ) ) ;
#25406=ORIENTED_EDGE ( 'NONE', *, *, #82007, .F. ) ;
#25429=ORIENTED_EDGE ( 'NONE', *, *, #71311, .T. ) ;
#25430=CIRCLE ( 'NONE', #57319, 89.89999999999997726 ) ;
#25457=CARTESIAN_POINT ( 'NONE',  ( 70.63919639214310564, 91.07499999999996021, -53.97512327982435210 ) ) ;
#25522=LINE ( 'NONE', #45938, #70101 ) ;
#25525=DIRECTION ( 'NONE',  ( 0.000000000000000000, 1.000000000000000000, 0.000000000000000000 ) ) ;
#25532=EDGE_CURVE ( 'NONE', #35189, #37391, #85070, .T. ) ;
#25556=DIRECTION ( 'NONE',  ( 0.7071067811865389130, -0.000000000000000000, 0.7071067811865561215 ) ) ;
#25577=CARTESIAN_POINT ( 'NONE',  ( -12.60000000000000142, 83.38334056604452371, 117.6834004267381601 ) ) ;
#25615=DIRECTION ( 'NONE',  ( 0.000000000000000000, -1.000000000000000000, 0.000000000000000000 ) ) ;
#25628=LINE ( 'NONE', #18362, #4746 ) ;
#25652=CARTESIAN_POINT ( 'NONE',  ( -215.9000000000000057, 3.174999999999999822, -41.27499999999999858 ) ) ;
#25657=CARTESIAN_POINT ( 'NONE',  ( -47.08008653354679041, 92.40823363359756115, 74.62285435386985455 ) ) ;
#25682=CARTESIAN_POINT ( 'NONE',  ( -487.2989999999999782, 6.038608028953049711, 90.48749999999999716 ) ) ;
#25685=VECTOR ( 'NONE', #20198, 1000.000000000000000 ) ;
#25703=ORIENTED_EDGE ( 'NONE', *, *, #17959, .T. ) ;
#25774=DIRECTION ( 'NONE',  ( 0.000000000000000000, -1.000000000000000000, 0.000000000000000000 ) ) ;
#25778=EDGE_CURVE ( 'NONE', #57892, #11788, #35271, .T. ) ;
#25797=CARTESIAN_POINT ( 'NONE',  ( -4.084829003145262760, 94.58238198110524309, 118.4862812673465982 ) ) ;
#25810=VECTOR ( 'NONE', #39467, 1000.000000000000000 ) ;
#25816=AXIS2_PLACEMENT_3D ( 'NONE', #52754, #39167, #67311 ) ;
#25824=CYLINDRICAL_SURFACE ( 'NONE', #44093, 4.762500000000002842 ) ;
#25833=ORIENTED_EDGE ( 'NONE', *, *, #45548, .F. ) ;
#25852=LINE ( 'NONE', #26733, #3207 ) ;
#25855=CARTESIAN_POINT ( 'NONE',  ( -458.3598257906459708, 60.32499999999999574, 3.174999999999999822 ) ) ;
#25858=ORIENTED_EDGE ( 'NONE', *, *, #22790, .F. ) ;
#25861=EDGE_LOOP ( 'NONE', ( #45234, #47434, #70563, #71310 ) ) ;
#25879=LINE ( 'NONE', #35814, #81996 ) ;
#25902=ORIENTED_EDGE ( 'NONE', *, *, #29712, .F. ) ;
#25951=CARTESIAN_POINT ( 'NONE',  ( -254.0000000000000000, 3.174999999999999822, -41.27499999999999858 ) ) ;
#25961=AXIS2_PLACEMENT_3D ( 'NONE', #20127, #122, #53259 ) ;
#25976=DIRECTION ( 'NONE',  ( -1.000000000000000000, 0.000000000000000000, 0.000000000000000000 ) ) ;
#25996=LINE ( 'NONE', #19184, #63122 ) ;
#26018=CARTESIAN_POINT ( 'NONE',  ( -254.0000000000000000, 104.7749999999999915, -41.27499999999999858 ) ) ;
#26041=VECTOR ( 'NONE', #65718, 1000.000000000000000 ) ;
#26070=ORIENTED_EDGE ( 'NONE', *, *, #22203, .T. ) ;
#26071=AXIS2_PLACEMENT_3D ( 'NONE', #4705, #80570, #12411 ) ;
#26091=DIRECTION ( 'NONE',  ( 0.000000000000000000, 0.000000000000000000, 1.000000000000000000 ) ) ;
#26116=CARTESIAN_POINT ( 'NONE',  ( -47.09267117624717969, 92.49156081278650277, 74.71343019242331707 ) ) ;
#26123=ORIENTED_EDGE ( 'NONE', *, *, #82096, .F. ) ;
#26129=CARTESIAN_POINT ( 'NONE',  ( -75.03318300175403976, 88.97500000000002274, 34.21687604822299988 ) ) ;
#26137=EDGE_LOOP ( 'NONE', ( #46916, #65584, #59502, #13760 ) ) ;
#26161=ORIENTED_EDGE ( 'NONE', *, *, #53648, .T. ) ;
#26196=FACE_BOUND ( 'NONE', #76152, .T. ) ;
#26216=LINE ( 'NONE', #19404, #38091 ) ;
#26219=ORIENTED_EDGE ( 'NONE', *, *, #9520, .F. ) ;
#26244=CARTESIAN_POINT ( 'NONE',  ( -8.382543579435365544, 92.09976689429159080, 118.2597275672832069 ) ) ;
#26261=ORIENTED_EDGE ( 'NONE', *, *, #48067, .T. ) ;
#26268=VERTEX_POINT ( 'NONE', #46251 ) ;
#26352=CARTESIAN_POINT ( 'NONE',  ( -47.02966122971776741, 101.5999999999999943, 76.61736725193563302 ) ) ;
#26385=ORIENTED_EDGE ( 'NONE', *, *, #51285, .T. ) ;
#26393=ADVANCED_FACE ( 'NONE', ( #67617 ), #5401, .F. ) ;
#26412=PLANE ( 'NONE',  #69413 ) ;
#26435=VECTOR ( 'NONE', #19841, 1000.000000000000000 ) ;
#26478=CARTESIAN_POINT ( 'NONE',  ( -8.325041732967005004, 92.04361142620588510, 118.0642879194596446 ) ) ;
#26480=ORIENTED_EDGE ( 'NONE', *, *, #62533, .T. ) ;
#26519=SURFACE_SIDE_STYLE ('',( #55086 ) ) ;
#26548=DIRECTION ( 'NONE',  ( 1.000000000000000000, -7.570719237730591757E-15, 0.000000000000000000 ) ) ;
#26563=DIRECTION ( 'NONE',  ( -0.000000000000000000, -1.000000000000000000, -0.000000000000000000 ) ) ;
#26575=EDGE_CURVE ( 'NONE', #14882, #24211, #46407, .T. ) ;
#26581=ADVANCED_FACE ( 'NONE', ( #66611 ), #65715, .T. ) ;
#26628=DIRECTION ( 'NONE',  ( 1.000000000000000000, 0.000000000000000000, 0.000000000000000000 ) ) ;
#26643=CARTESIAN_POINT ( 'NONE',  ( 69.63919639214307722, 92.07499999999998863, 53.63573739454427880 ) ) ;
#26676=DIRECTION ( 'NONE',  ( -0.000000000000000000, -1.000000000000000000, -0.000000000000000000 ) ) ;
#26681=EDGE_CURVE ( 'NONE', #74344, #19571, #18915, .T. ) ;
#26690=DIRECTION ( 'NONE',  ( 0.000000000000000000, 1.000000000000000000, 0.000000000000000000 ) ) ;
#26702=EDGE_CURVE ( 'NONE', #87213, #63160, #5855, .T. ) ;
#26714=EDGE_CURVE ( 'NONE', #55378, #13441, #71096, .T. ) ;
#26721=DIRECTION ( 'NONE',  ( 0.000000000000000000, -0.000000000000000000, -1.000000000000000000 ) ) ;
#26724=AXIS2_PLACEMENT_3D ( 'NONE', #43029, #57111, #30328 ) ;
#26725=CARTESIAN_POINT ( 'NONE',  ( 69.30528942165814499, 92.51192757647309861, 54.77470860734664626 ) ) ;
#26733=CARTESIAN_POINT ( 'NONE',  ( -446.0240000000000009, 104.7749999999999915, -1.387778780781445991E-14 ) ) ;
#26776=CARTESIAN_POINT ( 'NONE',  ( -487.2989999999999782, 100.8062500000000057, 94.61194598552329182 ) ) ;
#26777=VERTEX_POINT ( 'NONE', #28752 ) ;
#26792=ORIENTED_EDGE ( 'NONE', *, *, #61627, .F. ) ;
#26812=EDGE_CURVE ( 'NONE', #58138, #77202, #65064, .T. ) ;
#26816=ORIENTED_EDGE ( 'NONE', *, *, #37400, .F. ) ;
#26819=DIRECTION ( 'NONE',  ( 0.000000000000000000, 0.000000000000000000, -1.000000000000000000 ) ) ;
#26820=DIRECTION ( 'NONE',  ( 0.000000000000000000, 0.000000000000000000, -1.000000000000000000 ) ) ;
#26825=ORIENTED_EDGE ( 'NONE', *, *, #11656, .T. ) ;
#26837=CARTESIAN_POINT ( 'NONE',  ( -492.0614999999999668, 93.66249999999999432, 95.25000000000000000 ) ) ;
#26842=VERTEX_POINT ( 'NONE', #1948 ) ;
#26847=DIRECTION ( 'NONE',  ( 0.7071067811865500152, -0.7071067811865451302, 1.287852911526284856E-16 ) ) ;
#26865=CARTESIAN_POINT ( 'NONE',  ( -2.859109359865526390, 70.27181035201802217, 118.3221464644018255 ) ) ;
#26870=CARTESIAN_POINT ( 'NONE',  ( -487.2989999999999782, 89.53805401447691281, 18.25625000000039933 ) ) ;
#26895=ORIENTED_EDGE ( 'NONE', *, *, #16649, .T. ) ;
#26919=CARTESIAN_POINT ( 'NONE',  ( -47.11752803141010304, 65.68786680169236547, 108.7909173056707317 ) ) ;
#26923=ADVANCED_FACE ( 'NONE', ( #2397 ), #21956, .T. ) ;
#26926=CARTESIAN_POINT ( 'NONE',  ( -12.51814195203456137, 84.20263175503735908, 117.6922463100763423 ) ) ;
#26952=AXIS2_PLACEMENT_3D ( 'NONE', #60939, #25525, #24634 ) ;
#26969=ORIENTED_EDGE ( 'NONE', *, *, #70421, .T. ) ;
#26979=CARTESIAN_POINT ( 'NONE',  ( 0.000000000000000000, 92.07499999999998863, 87.89999999999994884 ) ) ;
#27035=DIRECTION ( 'NONE',  ( 1.000000000000000000, 0.000000000000000000, 0.000000000000000000 ) ) ;
#27037=EDGE_CURVE ( 'NONE', #16242, #23402, #13237, .T. ) ;
#27106=ORIENTED_EDGE ( 'NONE', *, *, #2860, .T. ) ;
#27127=EDGE_CURVE ( 'NONE', #11211, #76903, #47281, .T. ) ;
#27136=DIRECTION ( 'NONE',  ( 1.000000000000000000, 0.000000000000000000, 0.000000000000000000 ) ) ;
#27142=CLOSED_SHELL ( 'NONE', ( #14754, #8238, #4157, #63115, #76156, #76689 ) ) ;
#27181=AXIS2_PLACEMENT_3D ( 'NONE', #2918, #29730, #50603 ) ;
#27191=PLANE ( 'NONE',  #74435 ) ;
#27193=PLANE ( 'NONE',  #31118 ) ;
#27195=DIRECTION ( 'NONE',  ( -0.000000000000000000, 1.000000000000000000, -0.000000000000000000 ) ) ;
#27217=VECTOR ( 'NONE', #72022, 1000.000000000000000 ) ;
#27223=DIRECTION ( 'NONE',  ( 0.000000000000000000, 0.000000000000000000, -1.000000000000000000 ) ) ;
#27227=EDGE_CURVE ( 'NONE', #84439, #51309, #23216, .T. ) ;
#27300=ORIENTED_EDGE ( 'NONE', *, *, #7824, .T. ) ;
#27310=FACE_OUTER_BOUND ( 'NONE', #39446, .T. ) ;
#27320=ADVANCED_FACE ( 'NONE', ( #85877 ), #85440, .T. ) ;
#27336=CARTESIAN_POINT ( 'NONE',  ( -487.2989999999999782, 97.78694598552370110, 18.25625000000050235 ) ) ;
#27384=VERTEX_POINT ( 'NONE', #70443 ) ;
#27394=FACE_OUTER_BOUND ( 'NONE', #45409, .T. ) ;
#27412=DIRECTION ( 'NONE',  ( 0.000000000000000000, 1.000000000000000000, 0.000000000000000000 ) ) ;
#27450=AXIS2_PLACEMENT_3D ( 'NONE', #38812, #80175, #59251 ) ;
#27453=ORIENTED_EDGE ( 'NONE', *, *, #30296, .T. ) ;
#27455=DIRECTION ( 'NONE',  ( 0.000000000000000000, 1.000000000000000000, 0.000000000000000000 ) ) ;
#27492=VECTOR ( 'NONE', #15585, 1000.000000000000000 ) ;
#27496=DIRECTION ( 'NONE',  ( 0.000000000000000000, 1.000000000000000000, 0.000000000000000000 ) ) ;
#27497=EDGE_LOOP ( 'NONE', ( #77513, #69428, #21992, #36876, #77609, #58430 ) ) ;
#27498=ORIENTED_EDGE ( 'NONE', *, *, #19651, .T. ) ;
#27500=VECTOR ( 'NONE', #3157, 999.9999999999998863 ) ;
#27515=VERTEX_POINT ( 'NONE', #59911 ) ;
#27522=ADVANCED_FACE ( 'NONE', ( #66285 ), #24086, .F. ) ;
#27575=DIRECTION ( 'NONE',  ( 0.000000000000000000, 0.000000000000000000, 1.000000000000000000 ) ) ;
#27623=DIRECTION ( 'NONE',  ( 0.000000000000000000, -1.000000000000000000, 0.000000000000000000 ) ) ;
#27636=CARTESIAN_POINT ( 'NONE',  ( -479.3614999999999782, 10.16305401447644030, 97.63125000000000853 ) ) ;
#27642=CARTESIAN_POINT ( 'NONE',  ( -487.2989999999999782, 18.41194598552324990, 83.34375000000000000 ) ) ;
#27644=FACE_OUTER_BOUND ( 'NONE', #2843, .T. ) ;
#27649=( GEOMETRIC_REPRESENTATION_CONTEXT ( 3 ) GLOBAL_UNCERTAINTY_ASSIGNED_CONTEXT ( ( #72339 ) ) GLOBAL_UNIT_ASSIGNED_CONTEXT ( ( #81063, #6523, #47386 ) ) REPRESENTATION_CONTEXT ( 'NONE', 'WORKASPACE' ) );
#27654=ADVANCED_FACE ( 'NONE', ( #19491 ), #13570, .T. ) ;
#27659=ORIENTED_EDGE ( 'NONE', *, *, #244, .T. ) ;
#27677=DIRECTION ( 'NONE',  ( 1.000000000000000000, 0.000000000000000000, 0.000000000000000000 ) ) ;
#27688=DIRECTION ( 'NONE',  ( -1.000000000000000000, 0.000000000000000000, 0.000000000000000000 ) ) ;
#27712=EDGE_LOOP ( 'NONE', ( #62158, #46031, #26219, #69321 ) ) ;
#27721=AXIS2_PLACEMENT_3D ( 'NONE', #24547, #10029, #86775 ) ;
#27756=LINE ( 'NONE', #75471, #61111 ) ;
#27760=DIRECTION ( 'NONE',  ( -0.000000000000000000, -1.000000000000000000, -0.000000000000000000 ) ) ;
#27795=FACE_BOUND ( 'NONE', #20547, .T. ) ;
#27822=CARTESIAN_POINT ( 'NONE',  ( -446.0240000000000009, 53.97500000000000142, 50.79999999999999716 ) ) ;
#27824=VECTOR ( 'NONE', #77820, 1000.000000000000000 ) ;
#27835=ORIENTED_EDGE ( 'NONE', *, *, #51290, .F. ) ;
#27847=AXIS2_PLACEMENT_3D ( 'NONE', #74911, #13573, #41264 ) ;
#27849=VECTOR ( 'NONE', #32074, 1000.000000000000000 ) ;
#27853=ORIENTED_EDGE ( 'NONE', *, *, #34415, .F. ) ;
#27906=CARTESIAN_POINT ( 'NONE',  ( 70.63919639214310564, 65.60000000000000853, 0.000000000000000000 ) ) ;
#27915=VERTEX_POINT ( 'NONE', #9445 ) ;
#27919=CARTESIAN_POINT ( 'NONE',  ( 70.63919639214310564, 49.07499999999999574, -53.97512327982435210 ) ) ;
#27991=DIRECTION ( 'NONE',  ( 0.3387333329185071573, -0.3387333329185072683, 0.8777923776952267776 ) ) ;
#28007=CIRCLE ( 'NONE', #7718, 38.10000000000000142 ) ;
#28041=EDGE_CURVE ( 'NONE', #30366, #970, #87536, .T. ) ;
#28056=DIRECTION ( 'NONE',  ( 0.000000000000000000, 0.5000000000000087708, -0.8660254037844336006 ) ) ;
#28072=CARTESIAN_POINT ( 'NONE',  ( -487.2989999999999782, 18.41194598552320016, 97.63125000000000853 ) ) ;
#28087=DIRECTION ( 'NONE',  ( -1.000000000000000000, 0.000000000000000000, 0.000000000000000000 ) ) ;
#28128=CARTESIAN_POINT ( 'NONE',  ( -41.60202597009397607, 65.59999999999998010, 50.85338361873603219 ) ) ;
#28157=CONICAL_SURFACE ( 'NONE', #16571, 16.33514202138210791, 0.7853981633974517207 ) ;
#28168=CARTESIAN_POINT ( 'NONE',  ( 7.751770026801673374, 72.45555771672430012, 118.3043497398993082 ) ) ;
#28181=ORIENTED_EDGE ( 'NONE', *, *, #20376, .T. ) ;
#28185=ORIENTED_EDGE ( 'NONE', *, *, #38923, .F. ) ;
#28191=LINE ( 'NONE', #55879, #48074 ) ;
#28204=ORIENTED_EDGE ( 'NONE', *, *, #3639, .F. ) ;
#28244=CARTESIAN_POINT ( 'NONE',  ( 1.650257911361945773, 95.04836909505033304, 118.3452167253284131 ) ) ;
#28245=EDGE_LOOP ( 'NONE', ( #65445, #3877, #50025, #74584, #7129, #80021, #60266 ) ) ;
#28261=DIRECTION ( 'NONE',  ( 0.000000000000000000, 1.000000000000000000, 5.300584669389750404E-15 ) ) ;
#28265=ORIENTED_EDGE ( 'NONE', *, *, #74403, .T. ) ;
#28301=DIRECTION ( 'NONE',  ( -1.000000000000000000, 0.000000000000000000, 0.000000000000000000 ) ) ;
#28306=CARTESIAN_POINT ( 'NONE',  ( -50.35902679310718355, 54.97499999999996589, 27.95514712793348977 ) ) ;
#28332=DIRECTION ( 'NONE',  ( -1.000000000000000000, 0.000000000000000000, 0.000000000000000000 ) ) ;
#28349=ADVANCED_FACE ( 'NONE', ( #77944 ), #36455, .T. ) ;
#28376=ORIENTED_EDGE ( 'NONE', *, *, #65446, .T. ) ;
#28422=DIRECTION ( 'NONE',  ( 1.000000000000000000, 0.000000000000000000, 0.000000000000000000 ) ) ;
#28447=ORIENTED_EDGE ( 'NONE', *, *, #74106, .F. ) ;
#28457=VERTEX_POINT ( 'NONE', #30672 ) ;
#28488=AXIS2_PLACEMENT_3D ( 'NONE', #11070, #3820, #81042 ) ;
#28490=CARTESIAN_POINT ( 'NONE',  ( -546.0365000000000464, 53.97500000000000142, 88.90000000000000568 ) ) ;
#28501=DIRECTION ( 'NONE',  ( 1.000000000000000000, 0.000000000000000000, 0.000000000000000000 ) ) ;
#28505=VECTOR ( 'NONE', #11738, 1000.000000000000114 ) ;
#28506=ORIENTED_EDGE ( 'NONE', *, *, #72598, .T. ) ;
#28523=ORIENTED_EDGE ( 'NONE', *, *, #26681, .F. ) ;
#28530=VECTOR ( 'NONE', #11980, 1000.000000000000000 ) ;
#28559=ORIENTED_EDGE ( 'NONE', *, *, #57812, .F. ) ;
#28574=VECTOR ( 'NONE', #59422, 1000.000000000000000 ) ;
#28599=VECTOR ( 'NONE', #64002, 1000.000000000000114 ) ;
#28608=CIRCLE ( 'NONE', #89566, 10.41399999999997839 ) ;
#28624=CARTESIAN_POINT ( 'NONE',  ( 5.616470115748687597, 71.15184505290909556, 118.4234566822760542 ) ) ;
#28629=EDGE_LOOP ( 'NONE', ( #41179, #40955 ) ) ;
#28635=DIRECTION ( 'NONE',  ( 0.000000000000000000, 0.000000000000000000, 1.000000000000000000 ) ) ;
#28667=ADVANCED_FACE ( 'NONE', ( #55547 ), #28782, .T. ) ;
#28686=CARTESIAN_POINT ( 'NONE',  ( -17.54031676229692849, 65.59999999999998010, 43.71138335376673467 ) ) ;
#28707=CARTESIAN_POINT ( 'NONE',  ( 6.662635722923305082, 93.25222367490323450, 118.1688145635824441 ) ) ;
#28752=CARTESIAN_POINT ( 'NONE',  ( -479.3614999999999782, 21.43125000000029701, 15.23694598552314972 ) ) ;
#28757=EDGE_CURVE ( 'NONE', #77829, #71894, #37378, .T. ) ;
#28776=PLANE ( 'NONE',  #12384 ) ;
#28782=PLANE ( 'NONE',  #69910 ) ;
#28795=EDGE_LOOP ( 'NONE', ( #32115, #14674, #89902, #60095 ) ) ;
#28821=VECTOR ( 'NONE', #63352, 1000.000000000000000 ) ;
#28841=CYLINDRICAL_SURFACE ( 'NONE', #1256, 38.10000000000000142 ) ;
#28849=AXIS2_PLACEMENT_3D ( 'NONE', #49558, #20093, #89582 ) ;
#28870=CARTESIAN_POINT ( 'NONE',  ( -465.6921742093550165, 47.62500000000000000, -3.174999999999999822 ) ) ;
#28874=ORIENTED_EDGE ( 'NONE', *, *, #70130, .T. ) ;
#28884=DIRECTION ( 'NONE',  ( -0.000000000000000000, -1.000000000000000000, -0.000000000000000000 ) ) ;
#28886=CIRCLE ( 'NONE', #25961, 89.89999999999997726 ) ;
#28902=CARTESIAN_POINT ( 'NONE',  ( -24.20305689751608824, 53.97499999999997300, 74.96110745944689313 ) ) ;
#28908=DIRECTION ( 'NONE',  ( 0.000000000000000000, 0.000000000000000000, 1.000000000000000000 ) ) ;
#28911=EDGE_CURVE ( 'NONE', #9022, #36325, #48082, .T. ) ;
#28923=ORIENTED_EDGE ( 'NONE', *, *, #58349, .F. ) ;
#28934=CARTESIAN_POINT ( 'NONE',  ( -12.53570085554762237, 80.47189671605593730, 117.8914246743695458 ) ) ;
#28992=VECTOR ( 'NONE', #78771, 1000.000000000000114 ) ;
#29005=VECTOR ( 'NONE', #86634, 1000.000000000000000 ) ;
#29008=AXIS2_PLACEMENT_3D ( 'NONE', #39358, #49171, #7854 ) ;
#29058=CARTESIAN_POINT ( 'NONE',  ( 0.000000000000000000, 93.07500000000001705, 88.90000000000000568 ) ) ;
#29063=AXIS2_PLACEMENT_3D ( 'NONE', #15125, #16029, #57795 ) ;
#29064=EDGE_LOOP ( 'NONE', ( #69247, #25703, #77549, #13127 ) ) ;
#29073=AXIS2_PLACEMENT_3D ( 'NONE', #48043, #74878, #34423 ) ;
#29075=CARTESIAN_POINT ( 'NONE',  ( -254.0000000000000000, 53.97500000000000142, 50.79999999999999716 ) ) ;
#29117=CARTESIAN_POINT ( 'NONE',  ( -7.336232340149017261, 72.29773750292761747, 118.1289122150180475 ) ) ;
#29140=DIRECTION ( 'NONE',  ( 1.000000000000000000, 0.000000000000000000, 0.000000000000000000 ) ) ;
#29142=DIRECTION ( 'NONE',  ( 0.2884130866282236250, -0.7071067811865507924, -0.6456143519637524975 ) ) ;
#29175=EDGE_CURVE ( 'NONE', #60931, #28457, #49429, .T. ) ;
#29178=LINE ( 'NONE', #43684, #88350 ) ;
#29210=LINE ( 'NONE', #16030, #27492 ) ;
#29225=AXIS2_PLACEMENT_3D ( 'NONE', #5322, #5773, #62514 ) ;
#29247=ORIENTED_EDGE ( 'NONE', *, *, #4068, .F. ) ;
#29251=CARTESIAN_POINT ( 'NONE',  ( -546.0365000000000464, 53.97500000000000142, 50.79999999999999716 ) ) ;
#29253=AXIS2_PLACEMENT_3D ( 'NONE', #49454, #14967, #48544 ) ;
#29272=ORIENTED_EDGE ( 'NONE', *, *, #25093, .F. ) ;
#29304=ORIENTED_EDGE ( 'NONE', *, *, #22420, .T. ) ;
#29324=VECTOR ( 'NONE', #23553, 1000.000000000000000 ) ;
#29341=AXIS2_PLACEMENT_3D ( 'NONE', #13792, #28301, #77363 ) ;
#29374=VECTOR ( 'NONE', #17547, 1000.000000000000000 ) ;
#29379=CARTESIAN_POINT ( 'NONE',  ( -487.2989999999999782, 86.51875000000001137, 86.36305401447658880 ) ) ;
#29387=CARTESIAN_POINT ( 'NONE',  ( -54.20184508647076171, 54.02065945192997987, 70.80016487573695372 ) ) ;
#29389=VECTOR ( 'NONE', #4280, 1000.000000000000000 ) ;
#29418=FACE_OUTER_BOUND ( 'NONE', #39414, .T. ) ;
#29469=VERTEX_POINT ( 'NONE', #82101 ) ;
#29529=EDGE_LOOP ( 'NONE', ( #42284, #55389 ) ) ;
#29626=EDGE_LOOP ( 'NONE', ( #66803, #12552, #66185, #15590 ) ) ;
#29635=CIRCLE ( 'NONE', #61520, 20.00000000000000355 ) ;
#29649=UNCERTAINTY_MEASURE_WITH_UNIT (LENGTH_MEASURE( 1.000000000000000082E-05 ), #8131, 'distance_accuracy_value', 'NONE');
#29651=AXIS2_PLACEMENT_3D ( 'NONE', #55452, #20961, #76376 ) ;
#29661=DIRECTION ( 'NONE',  ( 0.000000000000000000, 0.000000000000000000, 1.000000000000000000 ) ) ;
#29664=DIRECTION ( 'NONE',  ( 0.4078776986755216494, 0.000000000000000000, -0.9130365726098601531 ) ) ;
#29712=EDGE_CURVE ( 'NONE', #7158, #52534, #13234, .T. ) ;
#29730=DIRECTION ( 'NONE',  ( 1.000000000000000000, 0.000000000000000000, 0.000000000000000000 ) ) ;
#29731=ORIENTED_EDGE ( 'NONE', *, *, #37538, .F. ) ;
#29737=LINE ( 'NONE', #70166, #28821 ) ;
#29769=ORIENTED_EDGE ( 'NONE', *, *, #12511, .F. ) ;
#29804=ADVANCED_FACE ( 'NONE', ( #44320 ), #86132, .T. ) ;
#29818=ORIENTED_EDGE ( 'NONE', *, *, #39206, .T. ) ;
#29846=VERTEX_POINT ( 'NONE', #73824 ) ;
#29868=DIRECTION ( 'NONE',  ( 1.000000000000000000, 0.000000000000000000, 0.000000000000000000 ) ) ;
#29879=DIRECTION ( 'NONE',  ( 0.000000000000000000, 0.000000000000000000, 1.000000000000000000 ) ) ;
#29909=EDGE_CURVE ( 'NONE', #47878, #74702, #43856, .T. ) ;
#29923=AXIS2_PLACEMENT_3D ( 'NONE', #25119, #81457, #4685 ) ;
#29929=CIRCLE ( 'NONE', #13961, 17.33514202138210081 ) ;
#29965=EDGE_LOOP ( 'NONE', ( #50367, #1905 ) ) ;
#29966=ORIENTED_EDGE ( 'NONE', *, *, #43724, .T. ) ;
#29982=AXIS2_PLACEMENT_3D ( 'NONE', #41417, #69147, #83680 ) ;
#30016=EDGE_CURVE ( 'NONE', #52044, #43910, #58224, .T. ) ;
#30055=CARTESIAN_POINT ( 'NONE',  ( 12.49830496249506240, 84.20078624585569571, 117.6942513177057776 ) ) ;
#30067=EDGE_LOOP ( 'NONE', ( #33419, #72852, #80735, #50681 ) ) ;
#30080=DIRECTION ( 'NONE',  ( 0.000000000000000000, 0.000000000000000000, -1.000000000000000000 ) ) ;
#30172=CARTESIAN_POINT ( 'NONE',  ( 70.63919639214310564, 49.07499999999999574, -33.74458626278666884 ) ) ;
#30174=ORIENTED_EDGE ( 'NONE', *, *, #71171, .T. ) ;
#30222=CARTESIAN_POINT ( 'NONE',  ( 70.63919639214310564, 65.60000000000000853, 95.21359708083839735 ) ) ;
#30296=EDGE_CURVE ( 'NONE', #50718, #55800, #25114, .T. ) ;
#30307=LINE ( 'NONE', #21712, #4590 ) ;
#30311=EDGE_LOOP ( 'NONE', ( #38766, #18780, #37354, #26385 ) ) ;
#30326=EDGE_CURVE ( 'NONE', #76187, #36750, #11867, .T. ) ;
#30328=DIRECTION ( 'NONE',  ( 0.000000000000000000, 0.000000000000000000, 1.000000000000000000 ) ) ;
#30358=DIRECTION ( 'NONE',  ( 0.4999999999999915623, -0.8660254037844433705, 0.000000000000000000 ) ) ;
#30366=VERTEX_POINT ( 'NONE', #31473 ) ;
#30374=( GEOMETRIC_REPRESENTATION_CONTEXT ( 3 ) GLOBAL_UNCERTAINTY_ASSIGNED_CONTEXT ( ( #37815 ) ) GLOBAL_UNIT_ASSIGNED_CONTEXT ( ( #41919, #57347, #14694 ) ) REPRESENTATION_CONTEXT ( 'NONE', 'WORKASPACE' ) );
#30432=CARTESIAN_POINT ( 'NONE',  ( -215.9000000000000057, 3.174999999999999822, -41.27499999999999858 ) ) ;
#30482=ADVANCED_FACE ( 'NONE', ( #20876 ), #7694, .F. ) ;
#30499=PLANE ( 'NONE',  #18439 ) ;
#30507=CARTESIAN_POINT ( 'NONE',  ( 1.652234655685276277, 70.03180882406793728, 118.3472113678285638 ) ) ;
#30549=VERTEX_POINT ( 'NONE', #38513 ) ;
#30560=AXIS2_PLACEMENT_3D ( 'NONE', #10519, #16899, #44578 ) ;
#30598=FACE_OUTER_BOUND ( 'NONE', #31869, .T. ) ;
#30645=LINE ( 'NONE', #38782, #4649 ) ;
#30672=CARTESIAN_POINT ( 'NONE',  ( 12.70000000000000107, 82.54999999999999716, 117.8738102209307641 ) ) ;
#30713=ADVANCED_FACE ( 'NONE', ( #39854 ), #40755, .F. ) ;
#30722=DIRECTION ( 'NONE',  ( 0.000000000000000000, 0.000000000000000000, 1.000000000000000000 ) ) ;
#30729=VECTOR ( 'NONE', #54914, 1000.000000000000227 ) ;
#30731=DIRECTION ( 'NONE',  ( 0.000000000000000000, -0.8660254037844392627, 0.4999999999999990008 ) ) ;
#30764=CARTESIAN_POINT ( 'NONE',  ( -487.2989999999999782, 93.66249999999999432, 85.72499999999999432 ) ) ;
#30784=CARTESIAN_POINT ( 'NONE',  ( -15.88716625750469902, 91.07499999999996021, -53.54073290201169044 ) ) ;
#30805=CIRCLE ( 'NONE', #9039, 1.524000000000001132 ) ;
#30808=CARTESIAN_POINT ( 'NONE',  ( 0.000000000000000000, 91.07499999999996021, 38.10000000000000142 ) ) ;
#30815=CARTESIAN_POINT ( 'NONE',  ( -48.02966122971777452, 100.5999999999999659, 106.4272185163641780 ) ) ;
#30857=EDGE_CURVE ( 'NONE', #77207, #74702, #57304, .T. ) ;
#30914=EDGE_LOOP ( 'NONE', ( #50730, #44456, #77968, #70221 ) ) ;
#30918=CARTESIAN_POINT ( 'NONE',  ( -487.2989999999999782, 18.41194598552324990, 83.34375000000000000 ) ) ;
#30923=ORIENTED_EDGE ( 'NONE', *, *, #9055, .F. ) ;
#30932=EDGE_CURVE ( 'NONE', #58319, #77842, #42980, .T. ) ;
#30941=CARTESIAN_POINT ( 'NONE',  ( 12.43699659993004403, 84.61172699943961106, 117.7007664268632112 ) ) ;
#30949=CARTESIAN_POINT ( 'NONE',  ( 0.8330848375387808202, 69.94999999999998863, 118.3559999999999803 ) ) ;
#30965=CARTESIAN_POINT ( 'NONE',  ( -41.60202597009397607, 65.59999999999998010, 50.85338361873603219 ) ) ;
#30995=CARTESIAN_POINT ( 'NONE',  ( -546.0365000000000464, 53.97500000000000142, 50.79999999999999716 ) ) ;
#31041=FACE_OUTER_BOUND ( 'NONE', #46523, .T. ) ;
#31055=ORIENTED_EDGE ( 'NONE', *, *, #32562, .F. ) ;
#31094=FACE_OUTER_BOUND ( 'NONE', #45078, .T. ) ;
#31118=AXIS2_PLACEMENT_3D ( 'NONE', #74902, #40815, #14473 ) ;
#31131=ADVANCED_FACE ( 'NONE', ( #11622 ), #54704, .F. ) ;
#31150=ORIENTED_EDGE ( 'NONE', *, *, #12848, .T. ) ;
#31153=PLANE ( 'NONE',  #1131 ) ;
#31183=DIRECTION ( 'NONE',  ( 0.000000000000000000, 0.000000000000000000, 1.000000000000000000 ) ) ;
#31186=CARTESIAN_POINT ( 'NONE',  ( -487.2989999999999782, 21.43125000000029701, 15.23694598552314972 ) ) ;
#31206=AXIS2_PLACEMENT_3D ( 'NONE', #31220, #25301, #11225 ) ;
#31220=CARTESIAN_POINT ( 'NONE',  ( -54.12775174896490427, 55.97500000000000142, 69.87310403134814862 ) ) ;
#31256=AXIS2_PLACEMENT_3D ( 'NONE', #88810, #26563, #20656 ) ;
#31278=VERTEX_POINT ( 'NONE', #54250 ) ;
#31302=ADVANCED_FACE ( 'NONE', ( #33841 ), #40654, .F. ) ;
#31338=CYLINDRICAL_SURFACE ( 'NONE', #77547, 11.17600000000001970 ) ;
#31363=EDGE_CURVE ( 'NONE', #54435, #11233, #55596, .T. ) ;
#31364=ORIENTED_EDGE ( 'NONE', *, *, #51285, .F. ) ;
#31376=FACE_OUTER_BOUND ( 'NONE', #67543, .T. ) ;
#31377=VERTEX_POINT ( 'NONE', #27919 ) ;
#31381=DIRECTION ( 'NONE',  ( 1.000000000000000000, 0.000000000000000000, 0.000000000000000000 ) ) ;
#31403=ORIENTED_EDGE ( 'NONE', *, *, #53197, .F. ) ;
#31411=ORIENTED_EDGE ( 'NONE', *, *, #51314, .T. ) ;
#31418=ORIENTED_EDGE ( 'NONE', *, *, #34820, .T. ) ;
#31422=VECTOR ( 'NONE', #4021, 1000.000000000000227 ) ;
#31425=ORIENTED_EDGE ( 'NONE', *, *, #83708, .T. ) ;
#31435=DIRECTION ( 'NONE',  ( -0.000000000000000000, -1.000000000000000000, -0.000000000000000000 ) ) ;
#31452=CARTESIAN_POINT ( 'NONE',  ( -47.02966122971774610, 92.07499999999998863, 74.26049396966043048 ) ) ;
#31454=DIRECTION ( 'NONE',  ( 1.000000000000000000, 0.000000000000000000, 0.000000000000000000 ) ) ;
#31472=FACE_OUTER_BOUND ( 'NONE', #27497, .T. ) ;
#31473=CARTESIAN_POINT ( 'NONE',  ( -487.2989999999999782, 22.53639197104660141, 90.48749999999999716 ) ) ;
#31475=CARTESIAN_POINT ( 'NONE',  ( -12.69999999999999574, 82.13551494250060614, 117.8738102209306930 ) ) ;
#31496=DIRECTION ( 'NONE',  ( 0.000000000000000000, 0.000000000000000000, 1.000000000000000000 ) ) ;
#31549=CARTESIAN_POINT ( 'NONE',  ( -47.02966122971774610, 92.07499999999998863, 74.26049396966043048 ) ) ;
#31581=LINE ( 'NONE', #24780, #16690 ) ;
#31631=CARTESIAN_POINT ( 'NONE',  ( -487.2989999999999782, 93.66249999999999432, 11.11250000000040217 ) ) ;
#31639=ORIENTED_EDGE ( 'NONE', *, *, #61882, .F. ) ;
#31684=CARTESIAN_POINT ( 'NONE',  ( -41.60202597009397607, 40.59999999999997300, 50.85338361873603219 ) ) ;
#31695=CARTESIAN_POINT ( 'NONE',  ( -240.5296158183964792, 14.28749999999982201, 85.72499999999999432 ) ) ;
#31711=CARTESIAN_POINT ( 'NONE',  ( -12.70000000000000462, 83.37936054969095778, 117.8738102209308067 ) ) ;
#31730=CARTESIAN_POINT ( 'NONE',  ( -487.2989999999999782, 85.41360802895360393, 11.11250000000036131 ) ) ;
#31735=EDGE_CURVE ( 'NONE', #83342, #72907, #74180, .T. ) ;
#31776=AXIS2_PLACEMENT_3D ( 'NONE', #79429, #44419, #87119 ) ;
#31797=EDGE_CURVE ( 'NONE', #21236, #1301, #59490, .T. ) ;
#31822=CARTESIAN_POINT ( 'NONE',  ( 12.70000000000000284, 83.38917085147761554, 117.8738102209307925 ) ) ;
#31824=EDGE_CURVE ( 'NONE', #41012, #55523, #82806, .T. ) ;
#31833=CARTESIAN_POINT ( 'NONE',  ( 5.590585941178334295, 71.22800506564998102, 118.2263554555544118 ) ) ;
#31839=ORIENTED_EDGE ( 'NONE', *, *, #41349, .T. ) ;
#31846=EDGE_CURVE ( 'NONE', #11788, #57892, #78178, .T. ) ;
#31866=ORIENTED_EDGE ( 'NONE', *, *, #983, .F. ) ;
#31869=EDGE_LOOP ( 'NONE', ( #35179, #87068, #66120, #72176 ) ) ;
#31879=ORIENTED_EDGE ( 'NONE', *, *, #32960, .T. ) ;
#31887=AXIS2_PLACEMENT_3D ( 'NONE', #23362, #11037, #38738 ) ;
#31888=CARTESIAN_POINT ( 'NONE',  ( 12.70000000000000107, 82.54999999999999716, 92.46299999999996544 ) ) ;
#31899=PLANE ( 'NONE',  #25816 ) ;
#31903=DIRECTION ( 'NONE',  ( 0.000000000000000000, 0.5000000000000087708, -0.8660254037844336006 ) ) ;
#31915=ORIENTED_EDGE ( 'NONE', *, *, #79178, .F. ) ;
#31939=CONICAL_SURFACE ( 'NONE', #82748, 16.33514202138212923, 0.7853981633974482790 ) ;
#31960=ORIENTED_EDGE ( 'NONE', *, *, #75155, .F. ) ;
#31962=ORIENTED_EDGE ( 'NONE', *, *, #20808, .T. ) ;
#31966=LINE ( 'NONE', #59659, #70278 ) ;
#32034=CIRCLE ( 'NONE', #58172, 4.762500000000001066 ) ;
#32041=VECTOR ( 'NONE', #76687, 1000.000000000000000 ) ;
#32074=DIRECTION ( 'NONE',  ( -0.4999999999999932832, 0.8660254037844424824, 0.000000000000000000 ) ) ;
#32078=ORIENTED_EDGE ( 'NONE', *, *, #34820, .F. ) ;
#32115=ORIENTED_EDGE ( 'NONE', *, *, #14953, .F. ) ;
#32153=ADVANCED_FACE ( 'NONE', ( #59966 ), #86814, .T. ) ;
#32155=CARTESIAN_POINT ( 'NONE',  ( -10.79024059098301080, 89.26081878472081144, 118.0641780253921098 ) ) ;
#32166=CARTESIAN_POINT ( 'NONE',  ( -479.3614999999999782, 7.143750000000280487, 15.23694598552305024 ) ) ;
#32187=ADVANCED_FACE ( 'NONE', ( #59076 ), #87700, .F. ) ;
#32227=ORIENTED_EDGE ( 'NONE', *, *, #43724, .F. ) ;
#32251=ORIENTED_EDGE ( 'NONE', *, *, #813, .F. ) ;
#32274=CARTESIAN_POINT ( 'NONE',  ( 1.232595164407830946E-29, 69.95000000000000284, 118.3560000000000088 ) ) ;
#32335=AXIS2_PLACEMENT_3D ( 'NONE', #12227, #19034, #4518 ) ;
#32345=CYLINDRICAL_SURFACE ( 'NONE', #71056, 17.33514202138210081 ) ;
#32397=EDGE_LOOP ( 'NONE', ( #53487, #42468, #77205, #47879, #82275 ) ) ;
#32411=FACE_OUTER_BOUND ( 'NONE', #76929, .T. ) ;
#32429=VECTOR ( 'NONE', #79769, 1000.000000000000000 ) ;
#32462=DIRECTION ( 'NONE',  ( 0.000000000000000000, -1.000000000000000000, -8.792068030499130893E-15 ) ) ;
#32512=FACE_OUTER_BOUND ( 'NONE', #84730, .T. ) ;
#32554=LINE ( 'NONE', #60260, #39883 ) ;
#32562=EDGE_CURVE ( 'NONE', #42067, #50592, #84062, .T. ) ;
#32572=EDGE_CURVE ( 'NONE', #16242, #7908, #44871, .T. ) ;
#32616=LINE ( 'NONE', #33957, #37234 ) ;
#32627=DIRECTION ( 'NONE',  ( 1.000000000000000000, 0.000000000000000000, 0.000000000000000000 ) ) ;
#32680=ADVANCED_FACE ( 'NONE', ( #87927 ), #52905, .F. ) ;
#32684=DIRECTION ( 'NONE',  ( 0.000000000000000000, 0.000000000000000000, 1.000000000000000000 ) ) ;
#32697=VERTEX_POINT ( 'NONE', #6600 ) ;
#32730=DIRECTION ( 'NONE',  ( 0.2884130866282246797, -0.7071067811865454633, -0.6456143519637579375 ) ) ;
#32735=VECTOR ( 'NONE', #87489, 1000.000000000000000 ) ;
#32749=VERTEX_POINT ( 'NONE', #49713 ) ;
#32766=DIRECTION ( 'NONE',  ( -1.000000000000000000, -0.000000000000000000, -0.000000000000000000 ) ) ;
#32780=CIRCLE ( 'NONE', #26952, 17.33514202138209370 ) ;
#32800=ORIENTED_EDGE ( 'NONE', *, *, #70300, .F. ) ;
#32911=CARTESIAN_POINT ( 'NONE',  ( -47.02966122971773899, 65.60000000000000853, 66.31971987082251019 ) ) ;
#32920=VECTOR ( 'NONE', #9018, 1000.000000000000114 ) ;
#32936=DIRECTION ( 'NONE',  ( -1.000000000000000000, 0.000000000000000000, 0.000000000000000000 ) ) ;
#32960=EDGE_CURVE ( 'NONE', #72800, #87961, #65586, .T. ) ;
#33032=EDGE_LOOP ( 'NONE', ( #61980, #51360, #56878, #77562 ) ) ;
#33035=AXIS2_PLACEMENT_3D ( 'NONE', #6892, #8246, #49554 ) ;
#33039=CARTESIAN_POINT ( 'NONE',  ( -47.02966122971776031, 65.60000000000000853, 108.8289304395572401 ) ) ;
#33073=VECTOR ( 'NONE', #36507, 1000.000000000000000 ) ;
#33088=ADVANCED_FACE ( 'NONE', ( #46458 ), #61436, .F. ) ;
#33154=ORIENTED_EDGE ( 'NONE', *, *, #14429, .F. ) ;
#33164=EDGE_CURVE ( 'NONE', #61703, #26268, #86964, .T. ) ;
#33175=ORIENTED_EDGE ( 'NONE', *, *, #39821, .F. ) ;
#33180=DIRECTION ( 'NONE',  ( -1.000000000000000000, 0.000000000000000000, 0.000000000000000000 ) ) ;
#33181=DIRECTION ( 'NONE',  ( 0.000000000000000000, 0.000000000000000000, -1.000000000000000000 ) ) ;
#33189=CARTESIAN_POINT ( 'NONE',  ( -544.5124999999999318, 53.97500000000000142, 88.90000000000000568 ) ) ;
#33225=VERTEX_POINT ( 'NONE', #5148 ) ;
#33241=CARTESIAN_POINT ( 'NONE',  ( 70.63919639214310564, 91.07499999999996021, 0.000000000000000000 ) ) ;
#33243=ORIENTED_EDGE ( 'NONE', *, *, #244, .F. ) ;
#33318=AXIS2_PLACEMENT_3D ( 'NONE', #24671, #79215, #52337 ) ;
#33334=EDGE_CURVE ( 'NONE', #10966, #46111, #49596, .T. ) ;
#33359=EDGE_CURVE ( 'NONE', #72100, #74526, #45638, .T. ) ;
#33419=ORIENTED_EDGE ( 'NONE', *, *, #8566, .F. ) ;
#33436=CARTESIAN_POINT ( 'NONE',  ( -487.2989999999999782, 101.9113919710471947, 11.11250000000054072 ) ) ;
#33444=CARTESIAN_POINT ( 'NONE',  ( -41.60202597009397607, 65.59999999999998010, 50.85338361873603219 ) ) ;
#33481=VERTEX_POINT ( 'NONE', #69617 ) ;
#33482=LINE ( 'NONE', #82110, #48549 ) ;
#33528=DIRECTION ( 'NONE',  ( 0.000000000000000000, 0.000000000000000000, -1.000000000000000000 ) ) ;
#33541=DIRECTION ( 'NONE',  ( 0.000000000000000000, 0.000000000000000000, 1.000000000000000000 ) ) ;
#33587=AXIS2_PLACEMENT_3D ( 'NONE', #69778, #71579, #15715 ) ;
#33595=CARTESIAN_POINT ( 'NONE',  ( -479.3614999999999782, 3.174999999999999822, -1.387778780781445991E-14 ) ) ;
#33631=DIRECTION ( 'NONE',  ( 0.000000000000000000, 0.000000000000000000, 1.000000000000000000 ) ) ;
#33642=LINE ( 'NONE', #12307, #80498 ) ;
#33681=EDGE_CURVE ( 'NONE', #43910, #22374, #33642, .T. ) ;
#33688=EDGE_CURVE ( 'NONE', #55859, #11211, #52880, .T. ) ;
#33689=DIRECTION ( 'NONE',  ( -0.000000000000000000, 1.000000000000000000, -0.000000000000000000 ) ) ;
#33708=CARTESIAN_POINT ( 'NONE',  ( -55.89999999999999858, 95.97500000000000853, 70.79999999999999716 ) ) ;
#33709=FACE_OUTER_BOUND ( 'NONE', #45669, .T. ) ;
#33712=AXIS2_PLACEMENT_3D ( 'NONE', #25682, #81575, #80667 ) ;
#33717=ORIENTED_EDGE ( 'NONE', *, *, #57812, .T. ) ;
#33778=FILL_AREA_STYLE ('',( #88760 ) ) ;
#33785=EDGE_CURVE ( 'NONE', #32749, #77919, #54451, .T. ) ;
#33819=CARTESIAN_POINT ( 'NONE',  ( 70.63919639214310564, 100.5999999999999659, 56.85413200336923012 ) ) ;
#33831=CARTESIAN_POINT ( 'NONE',  ( 0.000000000000000000, 82.54999999999999716, 92.46299999999996544 ) ) ;
#33841=FACE_OUTER_BOUND ( 'NONE', #43919, .T. ) ;
#33852=ORIENTED_EDGE ( 'NONE', *, *, #48411, .T. ) ;
#33863=ORIENTED_EDGE ( 'NONE', *, *, #18983, .T. ) ;
#33874=ORIENTED_EDGE ( 'NONE', *, *, #84353, .T. ) ;
#33889=DIRECTION ( 'NONE',  ( 0.000000000000000000, 1.000000000000000000, 1.056314557550181068E-14 ) ) ;
#33897=DIRECTION ( 'NONE',  ( 0.000000000000000000, 0.000000000000000000, -1.000000000000000000 ) ) ;
#33901=EDGE_CURVE ( 'NONE', #77829, #72800, #69060, .T. ) ;
#33912=CIRCLE ( 'NONE', #84707, 39.10000000000005116 ) ;
#33914=ORIENTED_EDGE ( 'NONE', *, *, #83532, .T. ) ;
#33939=CARTESIAN_POINT ( 'NONE',  ( 0.000000000000000000, 82.54999999999999716, 92.46299999999996544 ) ) ;
#33948=ORIENTED_EDGE ( 'NONE', *, *, #58355, .F. ) ;
#33957=CARTESIAN_POINT ( 'NONE',  ( -47.18030668273772221, 100.5999999999999659, 75.34738655934135920 ) ) ;
#33991=CARTESIAN_POINT ( 'NONE',  ( -492.0614999999999668, 14.28749999999982201, 95.25000000000000000 ) ) ;
#34000=DIRECTION ( 'NONE',  ( 0.000000000000000000, 0.000000000000000000, 1.000000000000000000 ) ) ;
#34005=DIRECTION ( 'NONE',  ( 0.000000000000000000, 0.000000000000000000, 1.000000000000000000 ) ) ;
#34058=PLANE ( 'NONE',  #74076 ) ;
#34064=EDGE_CURVE ( 'NONE', #57667, #54435, #86397, .T. ) ;
#34066=ORIENTED_EDGE ( 'NONE', *, *, #60157, .F. ) ;
#34068=ORIENTED_EDGE ( 'NONE', *, *, #37668, .F. ) ;
#34076=EDGE_CURVE ( 'NONE', #17700, #38989, #19663, .T. ) ;
#34118=LINE ( 'NONE', #76813, #40813 ) ;
#34120=VERTEX_POINT ( 'NONE', #12165 ) ;
#34156=DIRECTION ( 'NONE',  ( 0.000000000000000000, 7.536132396315209176E-17, -1.000000000000000000 ) ) ;
#34159=LINE ( 'NONE', #61863, #4337 ) ;
#34163=ORIENTED_EDGE ( 'NONE', *, *, #48192, .T. ) ;
#34168=DIRECTION ( 'NONE',  ( 1.000000000000000000, 0.000000000000000000, 0.000000000000000000 ) ) ;
#34169=AXIS2_PLACEMENT_3D ( 'NONE', #34487, #48993, #7689 ) ;
#34180=EDGE_CURVE ( 'NONE', #36750, #76187, #18167, .T. ) ;
#34188=DIRECTION ( 'NONE',  ( -1.000000000000000000, 0.000000000000000000, 0.000000000000000000 ) ) ;
#34195=ORIENTED_EDGE ( 'NONE', *, *, #64204, .T. ) ;
#34201=VECTOR ( 'NONE', #2769, 1000.000000000000000 ) ;
#34255=DIRECTION ( 'NONE',  ( 0.000000000000000000, 0.000000000000000000, -1.000000000000000000 ) ) ;
#34261=VECTOR ( 'NONE', #55256, 1000.000000000000000 ) ;
#34267=FACE_OUTER_BOUND ( 'NONE', #57597, .T. ) ;
#34285=EDGE_CURVE ( 'NONE', #42299, #77564, #82121, .T. ) ;
#34290=ORIENTED_EDGE ( 'NONE', *, *, #40048, .F. ) ;
#34298=ORIENTED_EDGE ( 'NONE', *, *, #6926, .T. ) ;
#34340=CARTESIAN_POINT ( 'NONE',  ( 70.63919639214310564, 100.5999999999999659, 0.000000000000000000 ) ) ;
#34343=VERTEX_POINT ( 'NONE', #40749 ) ;
#34372=ORIENTED_EDGE ( 'NONE', *, *, #62097, .T. ) ;
#34389=CIRCLE ( 'NONE', #86600, 4.762500000000000178 ) ;
#34390=DIRECTION ( 'NONE',  ( -0.9586846635221889512, 0.000000000000000000, 0.2844709403917162205 ) ) ;
#34409=FACE_OUTER_BOUND ( 'NONE', #36471, .T. ) ;
#34415=EDGE_CURVE ( 'NONE', #76903, #42953, #64471, .T. ) ;
#34423=DIRECTION ( 'NONE',  ( 0.000000000000000000, 0.000000000000000000, 1.000000000000000000 ) ) ;
#34430=CARTESIAN_POINT ( 'NONE',  ( -479.3614999999999782, 3.174999999999999822, 101.5999999999999943 ) ) ;
#34464=EDGE_CURVE ( 'NONE', #16194, #46234, #64671, .T. ) ;
#34484=DIRECTION ( 'NONE',  ( 0.000000000000000000, -5.300584669389750404E-15, 1.000000000000000000 ) ) ;
#34487=CARTESIAN_POINT ( 'NONE',  ( -47.18030668273772221, 100.5999999999999659, 75.34738655934135920 ) ) ;
#34498=EDGE_CURVE ( 'NONE', #26842, #18243, #17857, .T. ) ;
#34506=VERTEX_POINT ( 'NONE', #73256 ) ;
#34534=CARTESIAN_POINT ( 'NONE',  ( -254.0000000000000000, 14.28750000000026077, 11.11249999999970051 ) ) ;
#34540=CARTESIAN_POINT ( 'NONE',  ( 2.884098104289768205, 70.17475223863472422, 118.5216239073115929 ) ) ;
#34558=ORIENTED_EDGE ( 'NONE', *, *, #11600, .T. ) ;
#34584=FACE_OUTER_BOUND ( 'NONE', #83133, .T. ) ;
#34638=EDGE_CURVE ( 'NONE', #83829, #41798, #47782, .T. ) ;
#34643=DIRECTION ( 'NONE',  ( 0.000000000000000000, 0.000000000000000000, 1.000000000000000000 ) ) ;
#34644=ORIENTED_EDGE ( 'NONE', *, *, #65774, .T. ) ;
#34670=LINE ( 'NONE', #75121, #51418 ) ;
#34671=DIRECTION ( 'NONE',  ( 0.000000000000000000, 1.000000000000000000, 0.000000000000000000 ) ) ;
#34722=FACE_OUTER_BOUND ( 'NONE', #47461, .T. ) ;
#34776=VERTEX_POINT ( 'NONE', #77304 ) ;
#34805=PLANE ( 'NONE',  #29225 ) ;
#34820=EDGE_CURVE ( 'NONE', #40908, #19584, #54577, .T. ) ;
#34837=AXIS2_PLACEMENT_3D ( 'NONE', #61004, #13755, #82368 ) ;
#34896=FACE_OUTER_BOUND ( 'NONE', #76992, .T. ) ;
#34916=CARTESIAN_POINT ( 'NONE',  ( 70.63919639214310564, 100.5999999999999659, 56.85413200336923012 ) ) ;
#34926=ORIENTED_EDGE ( 'NONE', *, *, #7956, .T. ) ;
#34928=DIRECTION ( 'NONE',  ( 0.000000000000000000, 1.000000000000000000, 0.000000000000000000 ) ) ;
#34958=DIRECTION ( 'NONE',  ( 0.000000000000000000, -1.000000000000000000, 2.048885995248199879E-16 ) ) ;
#35023=CARTESIAN_POINT ( 'NONE',  ( -446.0240000000000009, 93.66249999999999432, 85.72499999999999432 ) ) ;
#35028=CYLINDRICAL_SURFACE ( 'NONE', #20371, 12.60000000000000142 ) ;
#35033=ADVANCED_FACE ( 'NONE', ( #2796 ), #17753, .F. ) ;
#35064=DIRECTION ( 'NONE',  ( 1.000000000000000000, 0.000000000000000000, 0.000000000000000000 ) ) ;
#35071=EDGE_CURVE ( 'NONE', #33225, #34343, #66203, .T. ) ;
#35090=ORIENTED_EDGE ( 'NONE', *, *, #56017, .F. ) ;
#35112=DIRECTION ( 'NONE',  ( -1.000000000000000000, 0.000000000000000000, 0.000000000000000000 ) ) ;
#35140=EDGE_CURVE ( 'NONE', #22043, #88630, #29929, .T. ) ;
#35145=CARTESIAN_POINT ( 'NONE',  ( -473.2019999999999982, 53.97500000000000142, -2.412999999999919876 ) ) ;
#35154=EDGE_LOOP ( 'NONE', ( #86037, #62216, #85338, #57217 ) ) ;
#35176=B_SPLINE_CURVE_WITH_KNOTS ( 'NONE', 3,
 ( #76281, #69472, #7248, #76732, #84006, #21780, #49448, #77188, #70364, #8139, #35829, #63546, #82225, #84908 ),
 .UNSPECIFIED., .F., .F.,
 ( 4, 2, 2, 2, 2, 2, 4 ),
 ( 0.000000000000000000, 0.0004142211558018930786, 0.0008284423116037861572, 0.001242663467405679236, 0.001656884623207572314, 0.002485326934811326813, 0.003313769246415081311 ),
 .UNSPECIFIED. ) ;
#35179=ORIENTED_EDGE ( 'NONE', *, *, #61243, .T. ) ;
#35189=VERTEX_POINT ( 'NONE', #26352 ) ;
#35243=CARTESIAN_POINT ( 'NONE',  ( -487.2989999999999782, 7.143750000000280487, 15.23694598552305024 ) ) ;
#35256=ORIENTED_EDGE ( 'NONE', *, *, #76557, .T. ) ;
#35271=CIRCLE ( 'NONE', #25087, 20.00000000000000355 ) ;
#35286=CARTESIAN_POINT ( 'NONE',  ( -487.2989999999999782, 93.66249999999999432, 82.23860802895320887 ) ) ;
#35287=ORIENTED_EDGE ( 'NONE', *, *, #35928, .T. ) ;
#35291=ORIENTED_EDGE ( 'NONE', *, *, #37400, .T. ) ;
#35314=CARTESIAN_POINT ( 'NONE',  ( -30.89999999999999858, 53.97500000000000142, 70.79999999999999716 ) ) ;
#35336=FACE_OUTER_BOUND ( 'NONE', #58497, .T. ) ;
#35351=ORIENTED_EDGE ( 'NONE', *, *, #53648, .F. ) ;
#35361=LINE ( 'NONE', #69901, #5464 ) ;
#35379=LINE ( 'NONE', #5911, #8059 ) ;
#35388=VECTOR ( 'NONE', #78713, 1000.000000000000000 ) ;
#35404=EDGE_CURVE ( 'NONE', #11233, #1571, #48816, .T. ) ;
#35432=ORIENTED_EDGE ( 'NONE', *, *, #73566, .F. ) ;
#35440=EDGE_CURVE ( 'NONE', #42953, #74494, #54610, .T. ) ;
#35444=ORIENTED_EDGE ( 'NONE', *, *, #72598, .F. ) ;
#35504=CARTESIAN_POINT ( 'NONE',  ( 5.580981516429890377, 93.85413957563092424, 118.2249067917183396 ) ) ;
#35524=ADVANCED_FACE ( 'NONE', ( #68928 ), #47565, .F. ) ;
#35581=DIRECTION ( 'NONE',  ( 0.000000000000000000, -0.8660254037844390407, 0.4999999999999995004 ) ) ;
#35594=DIRECTION ( 'NONE',  ( 0.000000000000000000, -1.000000000000000000, -8.792068030499130893E-15 ) ) ;
#35648=AXIS2_PLACEMENT_3D ( 'NONE', #30432, #79036, #9987 ) ;
#35683=DIRECTION ( 'NONE',  ( -0.000000000000000000, 1.000000000000000000, -0.000000000000000000 ) ) ;
#35696=CARTESIAN_POINT ( 'NONE',  ( -48.67264380398863466, 64.60000000000000853, 66.68100227564390536 ) ) ;
#35703=CARTESIAN_POINT ( 'NONE',  ( -55.89999999999999858, 53.97500000000000142, 70.79999999999999716 ) ) ;
#35739=ADVANCED_FACE ( 'NONE', ( #51594 ), #85710, .T. ) ;
#35744=LINE ( 'NONE', #44338, #51133 ) ;
#35749=DIRECTION ( 'NONE',  ( 0.000000000000000000, -1.000000000000000000, 0.000000000000000000 ) ) ;
#35756=EDGE_CURVE ( 'NONE', #83168, #43607, #45952, .T. ) ;
#35786=CARTESIAN_POINT ( 'NONE',  ( -487.2989999999999782, 10.16305401447645984, 83.34375000000000000 ) ) ;
#35792=ORIENTED_EDGE ( 'NONE', *, *, #19651, .F. ) ;
#35800=EDGE_LOOP ( 'NONE', ( #6378, #39229 ) ) ;
#35808=EDGE_LOOP ( 'NONE', ( #76493, #80141, #5614, #49706 ) ) ;
#35814=CARTESIAN_POINT ( 'NONE',  ( -12.60000000000000142, 82.54999999999999716, 89.46299999999996544 ) ) ;
#35815=LINE ( 'NONE', #63532, #21116 ) ;
#35821=EDGE_CURVE ( 'NONE', #82548, #16017, #14030, .T. ) ;
#35829=CARTESIAN_POINT ( 'NONE',  ( -75.64365119985745878, 54.20154546050554956, 30.80107733549443694 ) ) ;
#35853=CARTESIAN_POINT ( 'NONE',  ( -458.3598257906459708, 60.32499999999999574, -3.174999999999999822 ) ) ;
#35866=VERTEX_POINT ( 'NONE', #73839 ) ;
#35894=CARTESIAN_POINT ( 'NONE',  ( 61.00843881761244347, 49.07499999999999574, -33.74458626278666884 ) ) ;
#35906=ORIENTED_EDGE ( 'NONE', *, *, #34076, .T. ) ;
#35928=EDGE_CURVE ( 'NONE', #78144, #36708, #79788, .T. ) ;
#35996=CIRCLE ( 'NONE', #57777, 17.33514202138210791 ) ;
#36004=AXIS2_PLACEMENT_3D ( 'NONE', #75183, #32936, #67462 ) ;
#36007=VERTEX_POINT ( 'NONE', #59304 ) ;
#36022=PLANE ( 'NONE',  #13145 ) ;
#36085=PLANE ( 'NONE',  #54836 ) ;
#36090=DIRECTION ( 'NONE',  ( -1.000000000000000000, 0.000000000000000000, 0.000000000000000000 ) ) ;
#36110=CARTESIAN_POINT ( 'NONE',  ( 0.000000000000000000, 82.54999999999999716, 92.46299999999996544 ) ) ;
#36134=LINE ( 'NONE', #22080, #49305 ) ;
#36137=DIRECTION ( 'NONE',  ( 0.000000000000000000, 1.000000000000000000, 0.000000000000000000 ) ) ;
#36144=DIRECTION ( 'NONE',  ( 0.9130365726098601531, 0.000000000000000000, 0.4078776986755214828 ) ) ;
#36154=VECTOR ( 'NONE', #31435, 1000.000000000000000 ) ;
#36174=ADVANCED_FACE ( 'NONE', ( #58318 ), #57871, .T. ) ;
#36176=ORIENTED_EDGE ( 'NONE', *, *, #84353, .F. ) ;
#36189=DIRECTION ( 'NONE',  ( 0.000000000000000000, 0.000000000000000000, 1.000000000000000000 ) ) ;
#36211=EDGE_CURVE ( 'NONE', #72546, #31377, #22926, .T. ) ;
#36246=FACE_OUTER_BOUND ( 'NONE', #14856, .T. ) ;
#36278=FACE_OUTER_BOUND ( 'NONE', #62522, .T. ) ;
#36286=DIRECTION ( 'NONE',  ( -1.000000000000000000, 0.000000000000000000, 0.000000000000000000 ) ) ;
#36299=EDGE_LOOP ( 'NONE', ( #59383, #82039 ) ) ;
#36320=DIRECTION ( 'NONE',  ( 1.699132800883997481E-15, 0.000000000000000000, -1.000000000000000000 ) ) ;
#36325=VERTEX_POINT ( 'NONE', #9285 ) ;
#36335=FACE_OUTER_BOUND ( 'NONE', #86783, .T. ) ;
#36355=CIRCLE ( 'NONE', #66810, 16.33514202138210791 ) ;
#36372=DIRECTION ( 'NONE',  ( 0.000000000000000000, 0.000000000000000000, -1.000000000000000000 ) ) ;
#36384=DIRECTION ( 'NONE',  ( 1.000000000000000000, 0.000000000000000000, 0.000000000000000000 ) ) ;
#36385=ORIENTED_EDGE ( 'NONE', *, *, #42084, .F. ) ;
#36391=LINE ( 'NONE', #63640, #61746 ) ;
#36402=AXIS2_PLACEMENT_3D ( 'NONE', #78024, #28501, #55735 ) ;
#36439=CARTESIAN_POINT ( 'NONE',  ( 12.59999999999999964, 81.72717280875430390, 117.6834004267382028 ) ) ;
#36452=ORIENTED_EDGE ( 'NONE', *, *, #35440, .F. ) ;
#36455=TOROIDAL_SURFACE ( 'NONE', #33587, 10.00000000000000355, 10.00000000000000000 ) ;
#36460=DIRECTION ( 'NONE',  ( -1.821299053822143307E-16, 0.000000000000000000, 1.000000000000000000 ) ) ;
#36471=EDGE_LOOP ( 'NONE', ( #85678, #56540 ) ) ;
#36484=CARTESIAN_POINT ( 'NONE',  ( -487.2989999999999782, 85.41360802895360393, 11.11250000000036131 ) ) ;
#36487=DIRECTION ( 'NONE',  ( 0.000000000000000000, 0.000000000000000000, -1.000000000000000000 ) ) ;
#36507=DIRECTION ( 'NONE',  ( 1.000000000000000000, 0.000000000000000000, 0.000000000000000000 ) ) ;
#36631=LINE ( 'NONE', #42515, #83349 ) ;
#36681=EDGE_CURVE ( 'NONE', #75662, #86124, #79912, .T. ) ;
#36689=ORIENTED_EDGE ( 'NONE', *, *, #39535, .F. ) ;
#36705=LINE ( 'NONE', #43937, #89024 ) ;
#36708=VERTEX_POINT ( 'NONE', #4027 ) ;
#36711=ORIENTED_EDGE ( 'NONE', *, *, #55169, .T. ) ;
#36722=VERTEX_POINT ( 'NONE', #31730 ) ;
#36750=VERTEX_POINT ( 'NONE', #50379 ) ;
#36781=ORIENTED_EDGE ( 'NONE', *, *, #6288, .T. ) ;
#36792=CARTESIAN_POINT ( 'NONE',  ( -41.60202597009397607, 65.59999999999998010, 50.85338361873603219 ) ) ;
#36793=ORIENTED_EDGE ( 'NONE', *, *, #14957, .T. ) ;
#36795=CARTESIAN_POINT ( 'NONE',  ( 0.000000000000000000, 92.07499999999998863, 39.10000000000005116 ) ) ;
#36837=DIRECTION ( 'NONE',  ( 1.000000000000000000, 0.000000000000000000, 0.000000000000000000 ) ) ;
#36841=ORIENTED_EDGE ( 'NONE', *, *, #37538, .T. ) ;
#36864=CARTESIAN_POINT ( 'NONE',  ( 12.60000000000000142, 82.96121956631253624, 117.6834004267381744 ) ) ;
#36867=EDGE_CURVE ( 'NONE', #40115, #7001, #32616, .T. ) ;
#36875=CARTESIAN_POINT ( 'NONE',  ( 9.493161119239731605, 74.22443474232989047, 117.9761073818194603 ) ) ;
#36876=ORIENTED_EDGE ( 'NONE', *, *, #55411, .T. ) ;
#36892=VERTEX_POINT ( 'NONE', #81696 ) ;
#36929=PLANE ( 'NONE',  #63705 ) ;
#36942=FACE_OUTER_BOUND ( 'NONE', #78624, .T. ) ;
#36973=ADVANCED_FACE ( 'NONE', ( #34409 ), #77110, .T. ) ;
#36983=AXIS2_PLACEMENT_3D ( 'NONE', #81661, #25774, #13496 ) ;
#36996=CARTESIAN_POINT ( 'NONE',  ( -487.2989999999999782, 93.66249999999999432, 11.11250000000040217 ) ) ;
#36997=EDGE_CURVE ( 'NONE', #16194, #24603, #76652, .T. ) ;
#37030=CARTESIAN_POINT ( 'NONE',  ( -31.46309309085269845, 53.97500000000000142, 37.49170920442474397 ) ) ;
#37075=ORIENTED_EDGE ( 'NONE', *, *, #71031, .T. ) ;
#37080=CARTESIAN_POINT ( 'NONE',  ( -544.5124999999999318, 53.97500000000000142, 50.79999999999999716 ) ) ;
#37114=VECTOR ( 'NONE', #45533, 999.9999999999998863 ) ;
#37149=CARTESIAN_POINT ( 'NONE',  ( -487.2989999999999782, 100.8062500000000057, 86.36305401447658880 ) ) ;
#37180=AXIS2_PLACEMENT_3D ( 'NONE', #21117, #8843, #7486 ) ;
#37182=AXIS2_PLACEMENT_3D ( 'NONE', #10051, #65456, #18191 ) ;
#37206=ORIENTED_EDGE ( 'NONE', *, *, #81117, .F. ) ;
#37215=CARTESIAN_POINT ( 'NONE',  ( -41.60202597009397607, 40.59999999999997300, 50.85338361873603219 ) ) ;
#37234=VECTOR ( 'NONE', #88944, 1000.000000000000000 ) ;
#37280=AXIS2_PLACEMENT_3D ( 'NONE', #14023, #55770, #34005 ) ;
#37314=CARTESIAN_POINT ( 'NONE',  ( 11.74674901193918330, 87.43010368066354943, 117.9729399478468252 ) ) ;
#37324=VECTOR ( 'NONE', #702, 1000.000000000000000 ) ;
#37354=ORIENTED_EDGE ( 'NONE', *, *, #83334, .F. ) ;
#37358=AXIS2_PLACEMENT_3D ( 'NONE', #44513, #79969, #73119 ) ;
#37378=LINE ( 'NONE', #44172, #39418 ) ;
#37391=VERTEX_POINT ( 'NONE', #11067 ) ;
#37400=EDGE_CURVE ( 'NONE', #8859, #74897, #38770, .T. ) ;
#37416=CARTESIAN_POINT ( 'NONE',  ( -12.59749777234951651, 80.88611186001949704, 117.8848162280639684 ) ) ;
#37417=DIRECTION ( 'NONE',  ( -0.000000000000000000, 1.000000000000000000, -0.000000000000000000 ) ) ;
#37460=DIRECTION ( 'NONE',  ( 0.000000000000000000, -1.000000000000000000, 0.000000000000000000 ) ) ;
#37477=DIRECTION ( 'NONE',  ( -1.000000000000000000, 0.000000000000000000, 0.000000000000000000 ) ) ;
#37485=DIRECTION ( 'NONE',  ( -0.2884130866282256234, -0.7071067811865451302, 0.6456143519637580486 ) ) ;
#37505=AXIS2_PLACEMENT_3D ( 'NONE', #65865, #17292, #4097 ) ;
#37510=ORIENTED_EDGE ( 'NONE', *, *, #45576, .F. ) ;
#37516=CARTESIAN_POINT ( 'NONE',  ( -479.3614999999999782, 7.143750000000280487, 15.23694598552305024 ) ) ;
#37528=FACE_OUTER_BOUND ( 'NONE', #45380, .T. ) ;
#37538=EDGE_CURVE ( 'NONE', #15300, #56710, #59499, .T. ) ;
#37575=FACE_OUTER_BOUND ( 'NONE', #3487, .T. ) ;
#37581=DIRECTION ( 'NONE',  ( 0.000000000000000000, 1.000000000000000000, 0.000000000000000000 ) ) ;
#37586=LINE ( 'NONE', #57566, #7176 ) ;
#37622=EDGE_CURVE ( 'NONE', #47878, #67868, #35176, .T. ) ;
#37639=PLANE ( 'NONE',  #54703 ) ;
#37664=CIRCLE ( 'NONE', #7189, 4.762500000000002842 ) ;
#37668=EDGE_CURVE ( 'NONE', #8698, #86124, #43534, .T. ) ;
#37677=LINE ( 'NONE', #65377, #27500 ) ;
#37679=DIRECTION ( 'NONE',  ( 8.881784197001252323E-16, 0.000000000000000000, -1.000000000000000000 ) ) ;
#37697=DIRECTION ( 'NONE',  ( 0.000000000000000000, 0.000000000000000000, 1.000000000000000000 ) ) ;
#37700=CARTESIAN_POINT ( 'NONE',  ( -24.20305689751608824, 64.60000000000000853, 58.62596543806478877 ) ) ;
#37715=ADVANCED_FACE ( 'NONE', ( #24011 ), #37639, .T. ) ;
#37728=EDGE_CURVE ( 'NONE', #26842, #84840, #70820, .T. ) ;
#37734=CARTESIAN_POINT ( 'NONE',  ( -479.3614999999999782, 89.53805401447691281, 18.25625000000039933 ) ) ;
#37736=AXIS2_PLACEMENT_3D ( 'NONE', #74504, #38633, #80894 ) ;
#37765=CARTESIAN_POINT ( 'NONE',  ( 2.881808223710723649, 94.92563399540007651, 118.5216647685501670 ) ) ;
#37773=CARTESIAN_POINT ( 'NONE',  ( 6.314153984315725943, 71.61522187350405488, 118.1894436584348824 ) ) ;
#37779=ORIENTED_EDGE ( 'NONE', *, *, #42893, .F. ) ;
#37788=CARTESIAN_POINT ( 'NONE',  ( 0.000000000000000000, 92.07499999999998863, 0.000000000000000000 ) ) ;
#37812=VECTOR ( 'NONE', #19590, 1000.000000000000000 ) ;
#37815=UNCERTAINTY_MEASURE_WITH_UNIT (LENGTH_MEASURE( 1.000000000000000082E-05 ), #41919, 'distance_accuracy_value', 'NONE');
#37834=DIRECTION ( 'NONE',  ( -1.000000000000000000, 0.000000000000000000, 0.000000000000000000 ) ) ;
#37891=ADVANCED_FACE ( 'NONE', ( #62130 ), #75325, .F. ) ;
#37921=CARTESIAN_POINT ( 'NONE',  ( -454.6936515812919879, 53.97500000000000142, -3.174999999999999822 ) ) ;
#37937=DIRECTION ( 'NONE',  ( 1.000000000000000000, 0.000000000000000000, 0.000000000000000000 ) ) ;
#37970=VERTEX_POINT ( 'NONE', #1713 ) ;
#38054=ORIENTED_EDGE ( 'NONE', *, *, #30857, .T. ) ;
#38062=CYLINDRICAL_SURFACE ( 'NONE', #48187, 20.00000000000000355 ) ;
#38066=ORIENTED_EDGE ( 'NONE', *, *, #34076, .F. ) ;
#38070=CARTESIAN_POINT ( 'NONE',  ( 70.63919639214310564, 93.07500000000001705, 56.85413200336923012 ) ) ;
#38087=ORIENTED_EDGE ( 'NONE', *, *, #75396, .T. ) ;
#38091=VECTOR ( 'NONE', #82556, 1000.000000000000000 ) ;
#38112=EDGE_CURVE ( 'NONE', #15662, #55859, #72967, .T. ) ;
#38134=DIRECTION ( 'NONE',  ( 0.000000000000000000, 0.000000000000000000, -1.000000000000000000 ) ) ;
#38176=ORIENTED_EDGE ( 'NONE', *, *, #10088, .T. ) ;
#38201=CARTESIAN_POINT ( 'NONE',  ( 12.60000000000000142, 82.54999999999999716, 117.6834004267381744 ) ) ;
#38202=ORIENTED_EDGE ( 'NONE', *, *, #87592, .F. ) ;
#38256=DIRECTION ( 'NONE',  ( 1.000000000000000000, 0.000000000000000000, 0.000000000000000000 ) ) ;
#38265=DIRECTION ( 'NONE',  ( 0.000000000000000000, 0.000000000000000000, 1.000000000000000000 ) ) ;
#38287=ORIENTED_EDGE ( 'NONE', *, *, #3742, .F. ) ;
#38297=CARTESIAN_POINT ( 'NONE',  ( -7.746754343058400494, 72.45238928964013780, 118.3046374534493026 ) ) ;
#38303=ORIENTED_EDGE ( 'NONE', *, *, #1604, .T. ) ;
#38330=CARTESIAN_POINT ( 'NONE',  ( 69.63919639214310564, 101.5999999999999943, 94.70900412239863897 ) ) ;
#38361=CARTESIAN_POINT ( 'NONE',  ( -487.2989999999999782, 10.16305401447644030, 97.63125000000000853 ) ) ;
#38452=DIRECTION ( 'NONE',  ( -1.000000000000000000, 0.000000000000000000, 0.000000000000000000 ) ) ;
#38483=VECTOR ( 'NONE', #26091, 1000.000000000000000 ) ;
#38513=CARTESIAN_POINT ( 'NONE',  ( 1.232595164407830946E-29, 69.95000000000000284, 118.3560000000000088 ) ) ;
#38521=CARTESIAN_POINT ( 'NONE',  ( -11.00625354133475042, 88.90020661696165405, 118.0441705883949908 ) ) ;
#38541=FACE_BOUND ( 'NONE', #78517, .T. ) ;
#38598=ORIENTED_EDGE ( 'NONE', *, *, #19953, .F. ) ;
#38631=DIRECTION ( 'NONE',  ( -1.000000000000000000, 0.000000000000000000, 0.000000000000000000 ) ) ;
#38633=DIRECTION ( 'NONE',  ( -0.000000000000000000, -1.000000000000000000, -0.000000000000000000 ) ) ;
#38637=CARTESIAN_POINT ( 'NONE',  ( 7.394472951914207393, 92.88361795698580181, 118.3256787633386296 ) ) ;
#38639=EDGE_CURVE ( 'NONE', #74526, #19430, #6401, .T. ) ;
#38662=CARTESIAN_POINT ( 'NONE',  ( -487.2989999999999782, 93.66249999999999432, 90.48749999999999716 ) ) ;
#38672=CARTESIAN_POINT ( 'NONE',  ( -479.3614999999999782, 22.53639197104660141, 90.48749999999999716 ) ) ;
#38690=EDGE_CURVE ( 'NONE', #13441, #72100, #44668, .T. ) ;
#38712=ORIENTED_EDGE ( 'NONE', *, *, #82732, .F. ) ;
#38738=DIRECTION ( 'NONE',  ( 1.821299053822143307E-16, 0.000000000000000000, -1.000000000000000000 ) ) ;
#38742=CARTESIAN_POINT ( 'NONE',  ( -10.09803707135884210, 74.80381226467314093, 118.1260670069656271 ) ) ;
#38766=ORIENTED_EDGE ( 'NONE', *, *, #47399, .T. ) ;
#38767=EDGE_CURVE ( 'NONE', #9022, #14474, #23632, .T. ) ;
#38770=LINE ( 'NONE', #81039, #28530 ) ;
#38782=CARTESIAN_POINT ( 'NONE',  ( -479.3614999999999782, 18.41194598552324990, 83.34375000000000000 ) ) ;
#38786=LINE ( 'NONE', #52386, #29389 ) ;
#38799=FACE_OUTER_BOUND ( 'NONE', #45906, .T. ) ;
#38812=CARTESIAN_POINT ( 'NONE',  ( -492.0614999999999668, 14.28750000000026077, 11.11249999999970051 ) ) ;
#38844=CYLINDRICAL_SURFACE ( 'NONE', #737, 4.762500000000002842 ) ;
#38860=VECTOR ( 'NONE', #68645, 1000.000000000000000 ) ;
#38890=DIRECTION ( 'NONE',  ( 0.000000000000000000, -0.8660254037844351549, -0.5000000000000061062 ) ) ;
#38923=EDGE_CURVE ( 'NONE', #79764, #24976, #67622, .T. ) ;
#38945=VECTOR ( 'NONE', #33180, 1000.000000000000000 ) ;
#38947=ORIENTED_EDGE ( 'NONE', *, *, #82096, .T. ) ;
#38989=VERTEX_POINT ( 'NONE', #45810 ) ;
#39013=CARTESIAN_POINT ( 'NONE',  ( -30.86579703273522668, 53.97499999999997300, 73.54054752236280024 ) ) ;
#39036=ORIENTED_EDGE ( 'NONE', *, *, #28757, .F. ) ;
#39054=CARTESIAN_POINT ( 'NONE',  ( -254.0000000000000000, 93.66249999999999432, 11.11250000000040217 ) ) ;
#39060=VECTOR ( 'NONE', #21838, 1000.000000000000000 ) ;
#39069=EDGE_LOOP ( 'NONE', ( #28874, #59435, #80095, #73444 ) ) ;
#39164=CARTESIAN_POINT ( 'NONE',  ( -492.0614999999999668, 14.28750000000026077, 11.11249999999970051 ) ) ;
#39165=VECTOR ( 'NONE', #77347, 1000.000000000000000 ) ;
#39167=DIRECTION ( 'NONE',  ( 0.000000000000000000, 2.048885995248194949E-16, 1.000000000000000000 ) ) ;
#39196=ORIENTED_EDGE ( 'NONE', *, *, #31824, .F. ) ;
#39206=EDGE_CURVE ( 'NONE', #10945, #40908, #15137, .T. ) ;
#39208=EDGE_CURVE ( 'NONE', #51309, #16242, #15807, .T. ) ;
#39229=ORIENTED_EDGE ( 'NONE', *, *, #79184, .F. ) ;
#39257=CARTESIAN_POINT ( 'NONE',  ( -487.2989999999999782, 14.28749999999982201, 85.72499999999999432 ) ) ;
#39274=DIRECTION ( 'NONE',  ( 0.000000000000000000, -1.000000000000000000, 0.000000000000000000 ) ) ;
#39332=VERTEX_POINT ( 'NONE', #52070 ) ;
#39358=CARTESIAN_POINT ( 'NONE',  ( 0.000000000000000000, 91.07499999999996021, 0.000000000000000000 ) ) ;
#39393=CARTESIAN_POINT ( 'NONE',  ( -487.2989999999999782, 14.28750000000023945, 19.36139197104649767 ) ) ;
#39403=CARTESIAN_POINT ( 'NONE',  ( -76.76779673090611311, 55.97500000000000142, 30.90025125786759830 ) ) ;
#39414=EDGE_LOOP ( 'NONE', ( #21717, #2136, #66255, #76735 ) ) ;
#39418=VECTOR ( 'NONE', #11802, 1000.000000000000000 ) ;
#39423=CARTESIAN_POINT ( 'NONE',  ( -1.665381768328644485, 95.16753744185723463, 118.5470859077611863 ) ) ;
#39425=FACE_OUTER_BOUND ( 'NONE', #71556, .T. ) ;
#39437=CARTESIAN_POINT ( 'NONE',  ( -17.13243906362141900, 148.4450814996825443, 42.79834678115690849 ) ) ;
#39446=EDGE_LOOP ( 'NONE', ( #80944, #50607, #27659, #33852, #18246, #86569 ) ) ;
#39467=DIRECTION ( 'NONE',  ( 0.000000000000000000, 0.000000000000000000, -1.000000000000000000 ) ) ;
#39535=EDGE_CURVE ( 'NONE', #37970, #51377, #64422, .T. ) ;
#39559=DIRECTION ( 'NONE',  ( -1.000000000000000000, 0.000000000000000000, 0.000000000000000000 ) ) ;
#39575=DIRECTION ( 'NONE',  ( 0.000000000000000000, 6.920681583949466031E-15, -1.000000000000000000 ) ) ;
#39601=DIRECTION ( 'NONE',  ( -0.000000000000000000, 1.000000000000000000, -0.000000000000000000 ) ) ;
#39629=DIRECTION ( 'NONE',  ( 0.000000000000000000, -0.8660254037844387076, -0.4999999999999998890 ) ) ;
#39639=EDGE_CURVE ( 'NONE', #60931, #47557, #79014, .T. ) ;
#39651=ORIENTED_EDGE ( 'NONE', *, *, #35404, .T. ) ;
#39691=CARTESIAN_POINT ( 'NONE',  ( -479.3614999999999782, 6.038608028953039941, 90.48749999999999716 ) ) ;
#39761=CARTESIAN_POINT ( 'NONE',  ( -454.6936515812919879, 53.97500000000000142, 3.174999999999999822 ) ) ;
#39786=DIRECTION ( 'NONE',  ( -1.000000000000000000, 0.000000000000000000, 0.000000000000000000 ) ) ;
#39791=CARTESIAN_POINT ( 'NONE',  ( -492.0614999999999668, 14.28750000000026077, 6.349999999999710099 ) ) ;
#39792=DIRECTION ( 'NONE',  ( 6.938893903907227392E-16, 0.000000000000000000, -1.000000000000000000 ) ) ;
#39798=ORIENTED_EDGE ( 'NONE', *, *, #68772, .F. ) ;
#39821=EDGE_CURVE ( 'NONE', #40115, #60827, #77575, .T. ) ;
#39829=DIRECTION ( 'NONE',  ( 0.000000000000000000, 0.000000000000000000, 1.000000000000000000 ) ) ;
#39854=FACE_OUTER_BOUND ( 'NONE', #85201, .T. ) ;
#39883=VECTOR ( 'NONE', #18944, 1000.000000000000000 ) ;
#39884=VECTOR ( 'NONE', #9826, 1000.000000000000114 ) ;
#39891=CARTESIAN_POINT ( 'NONE',  ( -469.3583484187089994, 53.97500000000000142, 3.174999999999999822 ) ) ;
#39958=DIRECTION ( 'NONE',  ( -0.000000000000000000, 1.000000000000000000, -0.000000000000000000 ) ) ;
#39973=ORIENTED_EDGE ( 'NONE', *, *, #22203, .F. ) ;
#39975=CARTESIAN_POINT ( 'NONE',  ( 70.30580606644517161, 91.40839032569790845, -53.86233103605738393 ) ) ;
#39980=ORIENTED_EDGE ( 'NONE', *, *, #56428, .F. ) ;
#40011=VECTOR ( 'NONE', #68577, 1000.000000000000000 ) ;
#40043=EDGE_CURVE ( 'NONE', #77842, #88397, #34670, .T. ) ;
#40048=EDGE_CURVE ( 'NONE', #76657, #82662, #55089, .T. ) ;
#40051=DIRECTION ( 'NONE',  ( -1.000000000000000000, 0.000000000000000000, 0.000000000000000000 ) ) ;
#40087=VERTEX_POINT ( 'NONE', #39691 ) ;
#40095=CARTESIAN_POINT ( 'NONE',  ( -9.473967051880050505, 90.86722304825821084, 117.9765084014371865 ) ) ;
#40115=VERTEX_POINT ( 'NONE', #60580 ) ;
#40124=ORIENTED_EDGE ( 'NONE', *, *, #14429, .T. ) ;
#40160=ORIENTED_EDGE ( 'NONE', *, *, #87316, .F. ) ;
#40194=VECTOR ( 'NONE', #18177, 1000.000000000000000 ) ;
#40238=CARTESIAN_POINT ( 'NONE',  ( -24.20305689751608824, 54.97499999999995879, 75.96110745944689313 ) ) ;
#40252=CARTESIAN_POINT ( 'NONE',  ( -492.0614999999999668, 93.66249999999999432, 11.11250000000040217 ) ) ;
#40260=PLANE ( 'NONE',  #11441 ) ;
#40286=AXIS2_PLACEMENT_3D ( 'NONE', #49512, #89641, #55073 ) ;
#40345=ORIENTED_EDGE ( 'NONE', *, *, #85922, .F. ) ;
#40353=ADVANCED_FACE ( 'NONE', ( #48075 ), #85153, .T. ) ;
#40358=CARTESIAN_POINT ( 'NONE',  ( 69.63919639214307722, 92.07499999999998863, 53.63573739454427880 ) ) ;
#40368=ORIENTED_EDGE ( 'NONE', *, *, #76725, .F. ) ;
#40394=VECTOR ( 'NONE', #52949, 1000.000000000000000 ) ;
#40406=LINE ( 'NONE', #33595, #24039 ) ;
#40437=CARTESIAN_POINT ( 'NONE',  ( -41.60202597009397607, 53.97499999999997300, 50.85338361873603219 ) ) ;
#40444=ORIENTED_EDGE ( 'NONE', *, *, #42893, .T. ) ;
#40465=AXIS2_PLACEMENT_3D ( 'NONE', #71301, #8624, #9069 ) ;
#40504=CARTESIAN_POINT ( 'NONE',  ( -48.02966122971775320, 100.5999999999999659, -8.747637655308301746E-15 ) ) ;
#40562=FACE_OUTER_BOUND ( 'NONE', #66935, .T. ) ;
#40566=CONICAL_SURFACE ( 'NONE', #53571, 88.90000000000000568, 0.7853981633974621568 ) ;
#40613=LINE ( 'NONE', #68329, #78081 ) ;
#40616=EDGE_CURVE ( 'NONE', #64816, #12332, #85333, .T. ) ;
#40620=ORIENTED_EDGE ( 'NONE', *, *, #68160, .F. ) ;
#40636=ORIENTED_EDGE ( 'NONE', *, *, #9194, .T. ) ;
#40652=CARTESIAN_POINT ( 'NONE',  ( -240.5296158183964792, 14.28750000000026077, 15.87499999999969802 ) ) ;
#40654=PLANE ( 'NONE',  #25021 ) ;
#40658=EDGE_LOOP ( 'NONE', ( #87345, #27106 ) ) ;
#40661=AXIS2_PLACEMENT_3D ( 'NONE', #54396, #82609, #53950 ) ;
#40675=ORIENTED_EDGE ( 'NONE', *, *, #76363, .T. ) ;
#40706=CARTESIAN_POINT ( 'NONE',  ( -48.26476610531311451, 53.97499999999997300, 65.76796570303405076 ) ) ;
#40749=CARTESIAN_POINT ( 'NONE',  ( -254.0000000000000000, 93.66249999999999432, 85.72499999999999432 ) ) ;
#40755=CYLINDRICAL_SURFACE ( 'NONE', #45169, 12.70000000000000107 ) ;
#40812=CARTESIAN_POINT ( 'NONE',  ( -479.3614999999999782, 53.97500000000000142, 50.79999999999999716 ) ) ;
#40813=VECTOR ( 'NONE', #70455, 1000.000000000000000 ) ;
#40815=DIRECTION ( 'NONE',  ( 0.000000000000000000, -1.000000000000000000, -1.365923996832131856E-16 ) ) ;
#40862=CARTESIAN_POINT ( 'NONE',  ( -40.89999999999999858, 53.97500000000000142, 40.79999999999999716 ) ) ;
#40866=DIRECTION ( 'NONE',  ( 0.000000000000000000, -1.000000000000000000, 0.000000000000000000 ) ) ;
#40907=DIRECTION ( 'NONE',  ( 1.000000000000000000, 0.000000000000000000, 0.000000000000000000 ) ) ;
#40908=VERTEX_POINT ( 'NONE', #28902 ) ;
#40939=DIRECTION ( 'NONE',  ( -0.000000000000000000, 1.000000000000000000, -0.000000000000000000 ) ) ;
#40947=EDGE_CURVE ( 'NONE', #22043, #84439, #23442, .T. ) ;
#40955=ORIENTED_EDGE ( 'NONE', *, *, #5522, .T. ) ;
#40958=PLANE ( 'NONE',  #71573 ) ;
#40993=CARTESIAN_POINT ( 'NONE',  ( -7.690723789128298016, 92.56496522704115648, 118.1078823055163838 ) ) ;
#41012=VERTEX_POINT ( 'NONE', #67415 ) ;
#41081=DIRECTION ( 'NONE',  ( 1.000000000000000000, 0.000000000000000000, 0.000000000000000000 ) ) ;
#41179=ORIENTED_EDGE ( 'NONE', *, *, #63223, .T. ) ;
#41202=ORIENTED_EDGE ( 'NONE', *, *, #676, .F. ) ;
#41210=DIRECTION ( 'NONE',  ( 0.000000000000000000, 1.000000000000000000, 0.000000000000000000 ) ) ;
#41264=DIRECTION ( 'NONE',  ( 0.000000000000000000, 0.000000000000000000, 1.000000000000000000 ) ) ;
#41338=CARTESIAN_POINT ( 'NONE',  ( 6.710101316248270109, 71.75931113341763989, 118.3664676705691505 ) ) ;
#41344=EDGE_CURVE ( 'NONE', #15378, #1971, #61943, .T. ) ;
#41347=VECTOR ( 'NONE', #58365, 1000.000000000000000 ) ;
#41349=EDGE_CURVE ( 'NONE', #10009, #59609, #40613, .T. ) ;
#41368=ORIENTED_EDGE ( 'NONE', *, *, #62596, .T. ) ;
#41382=PLANE ( 'NONE',  #87906 ) ;
#41389=VECTOR ( 'NONE', #5563, 1000.000000000000114 ) ;
#41410=PLANE ( 'NONE',  #47264 ) ;
#41417=CARTESIAN_POINT ( 'NONE',  ( -41.60202597009397607, 76.06518036156089124, 50.85338361873603219 ) ) ;
#41452=EDGE_CURVE ( 'NONE', #14599, #51171, #66436, .T. ) ;
#41459=DIRECTION ( 'NONE',  ( -7.570719237730541270E-15, -1.000000000000000000, 0.000000000000000000 ) ) ;
#41476=FACE_BOUND ( 'NONE', #29965, .T. ) ;
#41576=FACE_BOUND ( 'NONE', #19885, .T. ) ;
#41592=FACE_BOUND ( 'NONE', #57950, .T. ) ;
#41601=AXIS2_PLACEMENT_3D ( 'NONE', #58967, #86255, #22702 ) ;
#41608=ORIENTED_EDGE ( 'NONE', *, *, #64708, .F. ) ;
#41616=AXIS2_PLACEMENT_3D ( 'NONE', #10232, #37937, #44284 ) ;
#41627=VECTOR ( 'NONE', #10712, 1000.000000000000000 ) ;
#41638=VECTOR ( 'NONE', #72213, 1000.000000000000000 ) ;
#41676=CARTESIAN_POINT ( 'NONE',  ( -446.0240000000000009, 3.174999999999999822, -1.387778780781445991E-14 ) ) ;
#41703=ORIENTED_EDGE ( 'NONE', *, *, #85234, .T. ) ;
#41706=AXIS2_PLACEMENT_3D ( 'NONE', #53235, #18750, #46435 ) ;
#41768=ORIENTED_EDGE ( 'NONE', *, *, #56860, .F. ) ;
#41776=AXIS2_PLACEMENT_3D ( 'NONE', #53160, #86386, #11415 ) ;
#41798=VERTEX_POINT ( 'NONE', #44021 ) ;
#41805=PLANE ( 'NONE',  #57732 ) ;
#41815=DIRECTION ( 'NONE',  ( 0.000000000000000000, 0.000000000000000000, -1.000000000000000000 ) ) ;
#41828=DIRECTION ( 'NONE',  ( 1.000000000000000000, 0.000000000000000000, 0.000000000000000000 ) ) ;
#41919=( LENGTH_UNIT ( ) NAMED_UNIT ( * ) SI_UNIT ( .MILLI., .METRE. ) );
#41927=DIRECTION ( 'NONE',  ( 0.000000000000000000, -1.000000000000000000, 1.682382052829014912E-15 ) ) ;
#41946=ORIENTED_EDGE ( 'NONE', *, *, #14847, .T. ) ;
#41958=AXIS2_PLACEMENT_3D ( 'NONE', #81073, #5652, #47400 ) ;
#41996=VERTEX_POINT ( 'NONE', #24772 ) ;
#42001=AXIS2_PLACEMENT_3D ( 'NONE', #61496, #20628, #61945 ) ;
#42022=CARTESIAN_POINT ( 'NONE',  ( -47.02966122971773189, 65.60000000000000853, 35.44631899411619003 ) ) ;
#42032=FACE_OUTER_BOUND ( 'NONE', #19574, .T. ) ;
#42036=LINE ( 'NONE', #7534, #1477 ) ;
#42044=AXIS2_PLACEMENT_3D ( 'NONE', #66505, #86531, #4294 ) ;
#42067=VERTEX_POINT ( 'NONE', #12039 ) ;
#42084=EDGE_CURVE ( 'NONE', #41012, #78672, #17946, .T. ) ;
#42122=EDGE_LOOP ( 'NONE', ( #15924, #12645, #41946, #41368 ) ) ;
#42131=FACE_OUTER_BOUND ( 'NONE', #33032, .T. ) ;
#42163=SHAPE_DEFINITION_REPRESENTATION ( #74302, #87903 ) ;
#42167=AXIS2_PLACEMENT_3D ( 'NONE', #12927, #18836, #67418 ) ;
#42199=AXIS2_PLACEMENT_3D ( 'NONE', #51757, #79505, #53529 ) ;
#42239=LINE ( 'NONE', #44024, #78439 ) ;
#42252=CARTESIAN_POINT ( 'NONE',  ( -446.0240000000000009, 104.7749999999999915, -1.387778780781445991E-14 ) ) ;
#42279=CARTESIAN_POINT ( 'NONE',  ( -48.02966122971777452, 65.60000000000000853, 106.4272185163641780 ) ) ;
#42284=ORIENTED_EDGE ( 'NONE', *, *, #6244, .F. ) ;
#42299=VERTEX_POINT ( 'NONE', #83321 ) ;
#42365=SHAPE_REPRESENTATION_RELATIONSHIP ( 'NONE' , 'NONE' ,  #87903, #88996 ) ;
#42368=CARTESIAN_POINT ( 'NONE',  ( -41.60202597009397607, 40.59999999999997300, 50.85338361873603219 ) ) ;
#42411=ORIENTED_EDGE ( 'NONE', *, *, #55498, .T. ) ;
#42417=DIRECTION ( 'NONE',  ( 0.000000000000000000, 0.000000000000000000, 1.000000000000000000 ) ) ;
#42430=CARTESIAN_POINT ( 'NONE',  ( 0.000000000000000000, 92.07499999999998863, 0.000000000000000000 ) ) ;
#42446=DIRECTION ( 'NONE',  ( 1.000000000000000000, 0.000000000000000000, 0.000000000000000000 ) ) ;
#42453=CARTESIAN_POINT ( 'NONE',  ( 70.63919639214310564, 91.07499999999996021, 53.63573739454427880 ) ) ;
#42468=ORIENTED_EDGE ( 'NONE', *, *, #4045, .T. ) ;
#42515=CARTESIAN_POINT ( 'NONE',  ( -487.2989999999999782, 101.9113919710471947, 11.11250000000054072 ) ) ;
#42533=CARTESIAN_POINT ( 'NONE',  ( -3.299561022378064479, 70.25802837517115051, 118.5128751897481436 ) ) ;
#42537=EDGE_CURVE ( 'NONE', #63160, #87213, #24502, .T. ) ;
#42550=PLANE ( 'NONE',  #5446 ) ;
#42552=DIRECTION ( 'NONE',  ( -1.000000000000000000, 0.000000000000000000, 0.000000000000000000 ) ) ;
#42570=CIRCLE ( 'NONE', #67226, 10.00000000000000178 ) ;
#42606=ORIENTED_EDGE ( 'NONE', *, *, #676, .T. ) ;
#42667=ORIENTED_EDGE ( 'NONE', *, *, #14935, .T. ) ;
#42671=DIRECTION ( 'NONE',  ( 0.000000000000000000, 1.000000000000000000, 0.000000000000000000 ) ) ;
#42775=CARTESIAN_POINT ( 'NONE',  ( -458.3598257906459708, 47.62500000000000000, 3.174999999999999822 ) ) ;
#42787=VECTOR ( 'NONE', #22565, 1000.000000000000000 ) ;
#42816=CARTESIAN_POINT ( 'NONE',  ( -492.0614999999999668, 93.66249999999999432, 85.72499999999999432 ) ) ;
#42842=CARTESIAN_POINT ( 'NONE',  ( -487.2989999999999782, 14.28750000000036025, 2.863608028952925100 ) ) ;
#42893=EDGE_CURVE ( 'NONE', #78995, #16194, #62224, .T. ) ;
#42900=B_SPLINE_CURVE_WITH_KNOTS ( 'NONE', 3,
 ( #89243, #47428, #54676, #61070, #26116, #25657, #74706, #6559, #13383, #82441 ),
 .UNSPECIFIED., .F., .F.,
 ( 4, 3, 3, 4 ),
 ( 0.000000000000000000, 0.0007422984837643878831, 0.001113447966056068956, 0.001484597482653254429 ),
 .UNSPECIFIED. ) ;
#42903=ORIENTED_EDGE ( 'NONE', *, *, #40048, .T. ) ;
#42904=ORIENTED_EDGE ( 'NONE', *, *, #51008, .T. ) ;
#42919=VECTOR ( 'NONE', #82460, 1000.000000000000114 ) ;
#42953=VERTEX_POINT ( 'NONE', #54351 ) ;
#42977=CARTESIAN_POINT ( 'NONE',  ( -0.4144131305978647761, 69.85000000000000853, 118.5560000000000258 ) ) ;
#42980=LINE ( 'NONE', #8498, #6101 ) ;
#42983=VECTOR ( 'NONE', #82467, 1000.000000000000000 ) ;
#42993=ORIENTED_EDGE ( 'NONE', *, *, #82007, .T. ) ;
#43001=EDGE_CURVE ( 'NONE', #46234, #19810, #5706, .T. ) ;
#43022=ORIENTED_EDGE ( 'NONE', *, *, #72944, .F. ) ;
#43029=CARTESIAN_POINT ( 'NONE',  ( -24.20305689751608824, 53.97499999999997300, 58.62596543806478877 ) ) ;
#43049=ADVANCED_FACE ( 'NONE', ( #20766 ), #57886, .T. ) ;
#43098=ORIENTED_EDGE ( 'NONE', *, *, #20808, .F. ) ;
#43134=CARTESIAN_POINT ( 'NONE',  ( 12.61749071809201439, 80.88423752776510867, 117.8827827373610688 ) ) ;
#43170=CARTESIAN_POINT ( 'NONE',  ( -10.91394553148466606, 76.24004728773776662, 117.8518844485520987 ) ) ;
#43287=DIRECTION ( 'NONE',  ( -0.9130365726098600421, 0.000000000000000000, -0.4078776986755215939 ) ) ;
#43290=ORIENTED_EDGE ( 'NONE', *, *, #84809, .F. ) ;
#43339=ORIENTED_EDGE ( 'NONE', *, *, #34498, .T. ) ;
#43355=ORIENTED_EDGE ( 'NONE', *, *, #25093, .T. ) ;
#43366=DIRECTION ( 'NONE',  ( -0.000000000000000000, 1.000000000000000000, -0.000000000000000000 ) ) ;
#43385=CIRCLE ( 'NONE', #4231, 50.79999999999999716 ) ;
#43397=VECTOR ( 'NONE', #82863, 1000.000000000000000 ) ;
#43418=VERTEX_POINT ( 'NONE', #83790 ) ;
#43422=DIRECTION ( 'NONE',  ( -0.2884130866282254013, 0.7071067811865455743, 0.6456143519637577155 ) ) ;
#43457=ORIENTED_EDGE ( 'NONE', *, *, #41344, .T. ) ;
#43490=DIRECTION ( 'NONE',  ( -1.000000000000000000, 0.000000000000000000, -0.000000000000000000 ) ) ;
#43508=ADVANCED_FACE ( 'NONE', ( #31041 ), #40566, .F. ) ;
#43509=ORIENTED_EDGE ( 'NONE', *, *, #18983, .F. ) ;
#43526=SURFACE_SIDE_STYLE ('',( #15407 ) ) ;
#43533=EDGE_CURVE ( 'NONE', #16628, #8809, #87008, .T. ) ;
#43534=LINE ( 'NONE', #30815, #28599 ) ;
#43555=EDGE_CURVE ( 'NONE', #66470, #57667, #59180, .T. ) ;
#43563=DIRECTION ( 'NONE',  ( 0.000000000000000000, 0.000000000000000000, -1.000000000000000000 ) ) ;
#43574=AXIS2_PLACEMENT_3D ( 'NONE', #60900, #89520, #12311 ) ;
#43607=VERTEX_POINT ( 'NONE', #10159 ) ;
#43609=CARTESIAN_POINT ( 'NONE',  ( -487.2989999999999782, 10.16305401447644030, 97.63125000000000853 ) ) ;
#43617=CARTESIAN_POINT ( 'NONE',  ( -12.27414673741744089, 79.67290841380474831, 117.7178608090033265 ) ) ;
#43666=CARTESIAN_POINT ( 'NONE',  ( 3.273557253446674142, 94.74519041223615545, 118.3134806149962088 ) ) ;
#43677=CARTESIAN_POINT ( 'NONE',  ( 10.70529764341858048, 75.89205320364979457, 117.8710853958748430 ) ) ;
#43684=CARTESIAN_POINT ( 'NONE',  ( -12.70000000000000107, 82.54999999999999716, 92.46299999999996544 ) ) ;
#43705=CARTESIAN_POINT ( 'NONE',  ( -48.02966122971776741, 65.60000000000000853, 75.53254848357481421 ) ) ;
#43724=EDGE_CURVE ( 'NONE', #75492, #9288, #37664, .T. ) ;
#43731=CARTESIAN_POINT ( 'NONE',  ( -254.0000000000000000, 104.7749999999999915, -41.27499999999999858 ) ) ;
#43763=VECTOR ( 'NONE', #61277, 999.9999999999998863 ) ;
#43765=AXIS2_PLACEMENT_3D ( 'NONE', #1965, #29661, #50540 ) ;
#43820=VECTOR ( 'NONE', #25264, 1000.000000000000114 ) ;
#43856=( BOUNDED_CURVE ( )  B_SPLINE_CURVE ( 3, ( #74281, #26129, #53797, #12502 ),
 .UNSPECIFIED., .F., .F. ) 
 B_SPLINE_CURVE_WITH_KNOTS ( ( 4, 4 ),
 ( 0.1001674211615598831, 3.041425232428233372 ),
 .UNSPECIFIED. ) 
 CURVE ( )  GEOMETRIC_REPRESENTATION_ITEM ( )  RATIONAL_B_SPLINE_CURVE ( ( 1.000000000000000000, 0.3999999999999999667, 0.3999999999999999667, 1.000000000000000000 ) ) 
 REPRESENTATION_ITEM ( '' )  );
#43858=ORIENTED_EDGE ( 'NONE', *, *, #62596, .F. ) ;
#43870=ORIENTED_EDGE ( 'NONE', *, *, #74595, .T. ) ;
#43886=EDGE_CURVE ( 'NONE', #10009, #72907, #34159, .T. ) ;
#43910=VERTEX_POINT ( 'NONE', #71399 ) ;
#43919=EDGE_LOOP ( 'NONE', ( #8650, #18868, #66672, #53431 ) ) ;
#43937=CARTESIAN_POINT ( 'NONE',  ( -472.4400000000000546, 53.97500000000000142, -3.174999999999999822 ) ) ;
#43940=ORIENTED_EDGE ( 'NONE', *, *, #64575, .T. ) ;
#44021=CARTESIAN_POINT ( 'NONE',  ( -479.3614999999999782, 93.66249999999999432, 98.73639197104678544 ) ) ;
#44024=CARTESIAN_POINT ( 'NONE',  ( -487.2989999999999782, 93.66249999999999432, 98.73639197104678544 ) ) ;
#44055=CIRCLE ( 'NONE', #57084, 88.90000000000000568 ) ;
#44057=EDGE_LOOP ( 'NONE', ( #26070, #74097, #76841, #10163 ) ) ;
#44062=CARTESIAN_POINT ( 'NONE',  ( -11.93200775504469391, 78.48097692672455139, 117.7530658574009976 ) ) ;
#44070=EDGE_CURVE ( 'NONE', #10702, #8698, #79821, .T. ) ;
#44093=AXIS2_PLACEMENT_3D ( 'NONE', #4932, #32627, #33528 ) ;
#44102=CARTESIAN_POINT ( 'NONE',  ( -240.5296158183964792, 93.66249999999999432, 95.25000000000000000 ) ) ;
#44104=CARTESIAN_POINT ( 'NONE',  ( 6.359898905133524849, 93.57403044202068543, 118.3873059837162742 ) ) ;
#44136=EDGE_LOOP ( 'NONE', ( #84138, #66535, #12642, #83265, #56812, #40675 ) ) ;
#44143=ADVANCED_FACE ( 'NONE', ( #4574 ), #31939, .T. ) ;
#44157=MECHANICAL_DESIGN_GEOMETRIC_PRESENTATION_REPRESENTATION('',(#23901),#80431);
#44172=CARTESIAN_POINT ( 'NONE',  ( -487.2989999999999782, 10.16305401447645984, 83.34375000000000000 ) ) ;
#44239=AXIS2_PLACEMENT_3D ( 'NONE', #11473, #53666, #46855 ) ;
#44269=DIRECTION ( 'NONE',  ( -0.9419738712670564507, -1.744347090500093949E-16, -0.3356862014592719157 ) ) ;
#44284=DIRECTION ( 'NONE',  ( 0.000000000000000000, 0.000000000000000000, -1.000000000000000000 ) ) ;
#44320=FACE_OUTER_BOUND ( 'NONE', #68826, .T. ) ;
#44338=CARTESIAN_POINT ( 'NONE',  ( -64.50026246089650783, 64.60000000000000853, 59.61038444174924678 ) ) ;
#44343=EDGE_CURVE ( 'NONE', #42299, #36892, #78408, .T. ) ;
#44405=LINE ( 'NONE', #78525, #20844 ) ;
#44411=EDGE_LOOP ( 'NONE', ( #50516, #18987, #63019, #89543 ) ) ;
#44419=DIRECTION ( 'NONE',  ( -0.000000000000000000, 1.000000000000000000, -0.000000000000000000 ) ) ;
#44423=DIRECTION ( 'NONE',  ( 0.000000000000000000, 0.000000000000000000, 1.000000000000000000 ) ) ;
#44436=B_SPLINE_CURVE_WITH_KNOTS ( 'NONE', 3,
 ( #76194, #6705, #61652, #54825 ),
 .UNSPECIFIED., .F., .F.,
 ( 4, 4 ),
 ( 0.000000000000000000, 0.001454274669798057921 ),
 .UNSPECIFIED. ) ;
#44451=CYLINDRICAL_SURFACE ( 'NONE', #41601, 4.762500000000002842 ) ;
#44456=ORIENTED_EDGE ( 'NONE', *, *, #12848, .F. ) ;
#44458=ORIENTED_EDGE ( 'NONE', *, *, #64050, .F. ) ;
#44476=DIRECTION ( 'NONE',  ( 0.000000000000000000, 0.000000000000000000, -1.000000000000000000 ) ) ;
#44513=CARTESIAN_POINT ( 'NONE',  ( 0.000000000000000000, 82.54999999999999716, 89.46299999999996544 ) ) ;
#44522=FACE_OUTER_BOUND ( 'NONE', #32397, .T. ) ;
#44550=CARTESIAN_POINT ( 'NONE',  ( 5.630981057377994148, 93.96377546238062450, 118.4246973091026973 ) ) ;
#44574=CARTESIAN_POINT ( 'NONE',  ( 70.63919639214310564, 65.60000000000000853, -53.97512327982435210 ) ) ;
#44578=DIRECTION ( 'NONE',  ( 0.000000000000000000, 0.000000000000000000, -1.000000000000000000 ) ) ;
#44579=ORIENTED_EDGE ( 'NONE', *, *, #48870, .F. ) ;
#44592=DIRECTION ( 'NONE',  ( 0.000000000000000000, 1.000000000000000000, 0.000000000000000000 ) ) ;
#44601=APPLICATION_CONTEXT ( 'automotive_design' ) ;
#44651=ADVANCED_FACE ( 'NONE', ( #39425 ), #18528, .F. ) ;
#44655=PLANE ( 'NONE',  #31887 ) ;
#44659=CARTESIAN_POINT ( 'NONE',  ( -10.78744120855129118, 75.83493809012784936, 118.0644293552432345 ) ) ;
#44668=CIRCLE ( 'NONE', #18541, 50.79999999999999716 ) ;
#44680=CIRCLE ( 'NONE', #46161, 87.89999999999994884 ) ;
#44769=CARTESIAN_POINT ( 'NONE',  ( 70.63919639214310564, 91.07499999999996021, 0.000000000000000000 ) ) ;
#44779=ORIENTED_EDGE ( 'NONE', *, *, #70745, .F. ) ;
#44792=ORIENTED_EDGE ( 'NONE', *, *, #10778, .F. ) ;
#44841=ORIENTED_EDGE ( 'NONE', *, *, #11342, .F. ) ;
#44862=VECTOR ( 'NONE', #6217, 1000.000000000000000 ) ;
#44871=CIRCLE ( 'NONE', #63690, 16.33514202138213633 ) ;
#44874=DIRECTION ( 'NONE',  ( 0.000000000000000000, 0.000000000000000000, -1.000000000000000000 ) ) ;
#44877=EDGE_CURVE ( 'NONE', #34343, #33225, #7378, .T. ) ;
#44887=DIRECTION ( 'NONE',  ( 0.4634479843259246556, 0.000000000000000000, 0.8861241255175470455 ) ) ;
#44919=ORIENTED_EDGE ( 'NONE', *, *, #925, .T. ) ;
#44923=ORIENTED_EDGE ( 'NONE', *, *, #20775, .T. ) ;
#44939=DIRECTION ( 'NONE',  ( 0.5773502691896305050, -0.5773502691896303940, -0.5773502691896164052 ) ) ;
#44968=CARTESIAN_POINT ( 'NONE',  ( -15.89999999999999680, 53.97500000000000142, 70.79999999999999716 ) ) ;
#44996=CARTESIAN_POINT ( 'NONE',  ( -254.0000000000000000, 53.97500000000000853, 101.5999999999999943 ) ) ;
#44999=FACE_BOUND ( 'NONE', #48168, .T. ) ;
#45014=EDGE_LOOP ( 'NONE', ( #87586, #71535, #47894, #7896 ) ) ;
#45054=CARTESIAN_POINT ( 'NONE',  ( 0.000000000000000000, 65.60000000000000853, 38.10000000000000142 ) ) ;
#45078=EDGE_LOOP ( 'NONE', ( #3793, #56875, #24490, #25429 ) ) ;
#45099=CARTESIAN_POINT ( 'NONE',  ( -487.2989999999999782, 14.28750000000026077, 11.11249999999970051 ) ) ;
#45133=CARTESIAN_POINT ( 'NONE',  ( 69.97242935852821688, 101.2667670336148689, 94.87759905963716278 ) ) ;
#45141=DIRECTION ( 'NONE',  ( 0.000000000000000000, -1.000000000000000000, -3.491483361109380094E-15 ) ) ;
#45169=AXIS2_PLACEMENT_3D ( 'NONE', #67123, #75292, #47107 ) ;
#45182=VECTOR ( 'NONE', #80728, 999.9999999999998863 ) ;
#45195=EDGE_CURVE ( 'NONE', #31278, #8470, #1785, .T. ) ;
#45209=DIRECTION ( 'NONE',  ( 1.000000000000000000, 0.000000000000000000, 0.000000000000000000 ) ) ;
#45234=ORIENTED_EDGE ( 'NONE', *, *, #2860, .F. ) ;
#45246=LINE ( 'NONE', #72966, #27849 ) ;
#45301=DIRECTION ( 'NONE',  ( 0.000000000000000000, 0.000000000000000000, 1.000000000000000000 ) ) ;
#45305=ORIENTED_EDGE ( 'NONE', *, *, #74403, .F. ) ;
#45311=DIRECTION ( 'NONE',  ( -1.000000000000000000, 0.000000000000000000, 0.000000000000000000 ) ) ;
#45313=AXIS2_PLACEMENT_3D ( 'NONE', #12566, #47505, #13017 ) ;
#45324=CARTESIAN_POINT ( 'NONE',  ( -12.27294214581303500, 85.84208941621251654, 117.9191027095085218 ) ) ;
#45336=FACE_OUTER_BOUND ( 'NONE', #42122, .T. ) ;
#45365=LINE ( 'NONE', #66257, #41638 ) ;
#45379=CARTESIAN_POINT ( 'NONE',  ( -46.74837461823508278, 65.31871338851736652, -44.28436222200497241 ) ) ;
#45380=EDGE_LOOP ( 'NONE', ( #6427, #33175, #70892, #72650 ) ) ;
#45384=EDGE_LOOP ( 'NONE', ( #57117, #7564, #78992, #11405, #65365 ) ) ;
#45409=EDGE_LOOP ( 'NONE', ( #84225, #50404, #12166, #19128 ) ) ;
#45428=VECTOR ( 'NONE', #36460, 1000.000000000000000 ) ;
#45431=VERTEX_POINT ( 'NONE', #59124 ) ;
#45436=CARTESIAN_POINT ( 'NONE',  ( 12.26894765557485023, 85.85687052802856556, 117.9195186832830871 ) ) ;
#45443=CARTESIAN_POINT ( 'NONE',  ( 3.260455919141270087, 70.37212065169552488, 118.3117458384234624 ) ) ;
#45446=CARTESIAN_POINT ( 'NONE',  ( -30.86579703273522668, 65.60000000000000853, 73.54054752236280024 ) ) ;
#45455=DIRECTION ( 'NONE',  ( 0.000000000000000000, 0.000000000000000000, -1.000000000000000000 ) ) ;
#45491=CYLINDRICAL_SURFACE ( 'NONE', #65570, 38.10000000000000142 ) ;
#45508=FACE_OUTER_BOUND ( 'NONE', #511, .T. ) ;
#45524=ORIENTED_EDGE ( 'NONE', *, *, #40616, .F. ) ;
#45533=DIRECTION ( 'NONE',  ( 0.000000000000000000, -0.8660254037844390407, 0.4999999999999995004 ) ) ;
#45548=EDGE_CURVE ( 'NONE', #78672, #36722, #27756, .T. ) ;
#45562=ORIENTED_EDGE ( 'NONE', *, *, #2024, .T. ) ;
#45576=EDGE_CURVE ( 'NONE', #1971, #64816, #28191, .T. ) ;
#45599=CARTESIAN_POINT ( 'NONE',  ( -487.2989999999999782, 86.51875000000001137, 94.61194598552339130 ) ) ;
#45618=ORIENTED_EDGE ( 'NONE', *, *, #88880, .T. ) ;
#45638=CIRCLE ( 'NONE', #87752, 50.79999999999999716 ) ;
#45645=LINE ( 'NONE', #15857, #74773 ) ;
#45669=EDGE_LOOP ( 'NONE', ( #84520, #64485, #59608, #59778, #59795 ) ) ;
#45761=VECTOR ( 'NONE', #16524, 1000.000000000000000 ) ;
#45763=AXIS2_PLACEMENT_3D ( 'NONE', #81228, #67119, #24896 ) ;
#45766=CARTESIAN_POINT ( 'NONE',  ( -7.735768046436663603, 92.63082225456683716, 118.3037957712300283 ) ) ;
#45779=LINE ( 'NONE', #39437, #28574 ) ;
#45810=CARTESIAN_POINT ( 'NONE',  ( 50.42303506447345285, 65.60000000000000853, -73.21698938693724301 ) ) ;
#45871=DIRECTION ( 'NONE',  ( 0.000000000000000000, 0.000000000000000000, -1.000000000000000000 ) ) ;
#45882=LINE ( 'NONE', #87698, #60694 ) ;
#45884=CARTESIAN_POINT ( 'NONE',  ( -487.2989999999999782, 97.78694598552370110, 18.25625000000050235 ) ) ;
#45896=EDGE_LOOP ( 'NONE', ( #51041, #32251, #84712, #10338 ) ) ;
#45906=EDGE_LOOP ( 'NONE', ( #6917, #50104, #81473, #59531 ) ) ;
#45938=CARTESIAN_POINT ( 'NONE',  ( -254.0000000000000000, 3.174999999999999822, -41.27499999999999858 ) ) ;
#45952=CIRCLE ( 'NONE', #6823, 50.79999999999999716 ) ;
#45982=CARTESIAN_POINT ( 'NONE',  ( -487.2989999999999782, 100.8062500000000057, 86.36305401447658880 ) ) ;
#45994=CARTESIAN_POINT ( 'NONE',  ( -48.02966122971776741, 91.07499999999996021, 74.26049396966043048 ) ) ;
#46031=ORIENTED_EDGE ( 'NONE', *, *, #68038, .F. ) ;
#46107=VECTOR ( 'NONE', #79323, 1000.000000000000114 ) ;
#46111=VERTEX_POINT ( 'NONE', #6314 ) ;
#46113=CARTESIAN_POINT ( 'NONE',  ( 70.63919639214310564, 65.60000000000000853, -33.74458626278666884 ) ) ;
#46161=AXIS2_PLACEMENT_3D ( 'NONE', #42430, #70154, #7926 ) ;
#46165=ADVANCED_FACE ( 'NONE', ( #20405 ), #48076, .F. ) ;
#46166=FACE_OUTER_BOUND ( 'NONE', #69542, .T. ) ;
#46234=VERTEX_POINT ( 'NONE', #62618 ) ;
#46248=ORIENTED_EDGE ( 'NONE', *, *, #4194, .F. ) ;
#46250=EDGE_CURVE ( 'NONE', #9288, #75492, #62673, .T. ) ;
#46251=CARTESIAN_POINT ( 'NONE',  ( -492.0614999999999668, 14.28749999999982201, 95.25000000000000000 ) ) ;
#46279=VECTOR ( 'NONE', #415, 1000.000000000000000 ) ;
#46310=EDGE_CURVE ( 'NONE', #34506, #16953, #4645, .T. ) ;
#46316=EDGE_LOOP ( 'NONE', ( #12377, #4367, #8179, #11150 ) ) ;
#46321=DIRECTION ( 'NONE',  ( 0.000000000000000000, 1.000000000000000000, 0.000000000000000000 ) ) ;
#46358=ORIENTED_EDGE ( 'NONE', *, *, #37728, .F. ) ;
#46359=DIRECTION ( 'NONE',  ( 0.000000000000000000, 0.000000000000000000, 1.000000000000000000 ) ) ;
#46361=ORIENTED_EDGE ( 'NONE', *, *, #34180, .T. ) ;
#46373=CARTESIAN_POINT ( 'NONE',  ( -492.0614999999999668, 14.28750000000026077, 11.11249999999970051 ) ) ;
#46407=CIRCLE ( 'NONE', #81272, 50.79999999999999716 ) ;
#46435=DIRECTION ( 'NONE',  ( 0.000000000000000000, 0.000000000000000000, 1.000000000000000000 ) ) ;
#46438=CARTESIAN_POINT ( 'NONE',  ( -254.0000000000000000, 14.28750000000026077, 15.87499999999969802 ) ) ;
#46458=FACE_OUTER_BOUND ( 'NONE', #2600, .T. ) ;
#46462=VECTOR ( 'NONE', #11914, 1000.000000000000000 ) ;
#46471=FACE_OUTER_BOUND ( 'NONE', #75204, .T. ) ;
#46493=CARTESIAN_POINT ( 'NONE',  ( -487.2989999999999782, 100.8062500000000057, 94.61194598552329182 ) ) ;
#46520=AXIS2_PLACEMENT_3D ( 'NONE', #89167, #28261, #55956 ) ;
#46523=EDGE_LOOP ( 'NONE', ( #426, #18771, #73568, #35792 ) ) ;
#46524=B_SPLINE_CURVE_WITH_KNOTS ( 'NONE', 3,
 ( #68214, #5996, #89104, #26865, #54543, #20062, #47742, #50437, #49982, #29117, #78632, #23225, #77721, #15499, #70911, #22308, #43170, #23656, #1863, #44062, #58157, #43617, #8683, #65423, #71797 ),
 .UNSPECIFIED., .F., .F.,
 ( 4, 2, 2, 2, 2, 2, 2, 2, 2, 1, 2, 2, 4 ),
 ( 0.05913659445472881082, 0.06159867070730776911, 0.06282970883359724479, 0.06406074695988672740, 0.06652282321246567875, 0.06775386133875516137, 0.06898489946504463011, 0.07144697571762360921, 0.07267801384391310571, 0.07390905197020260220, 0.07514009009649209869, 0.07637112822278158131, 0.07883320447536057429 ),
 .UNSPECIFIED. ) ;
#46532=LINE ( 'NONE', #75613, #49941 ) ;
#46536=EDGE_CURVE ( 'NONE', #67868, #57892, #74361, .T. ) ;
#46565=VECTOR ( 'NONE', #49994, 1000.000000000000000 ) ;
#46594=EDGE_CURVE ( 'NONE', #88352, #72160, #18946, .T. ) ;
#46624=CARTESIAN_POINT ( 'NONE',  ( 70.63919639214310564, 93.07500000000001705, 56.85413200336923012 ) ) ;
#46637=PLANE ( 'NONE',  #18618 ) ;
#46640=DIRECTION ( 'NONE',  ( 1.000000000000000000, 0.000000000000000000, 0.000000000000000000 ) ) ;
#46646=ORIENTED_EDGE ( 'NONE', *, *, #85627, .F. ) ;
#46647=ORIENTED_EDGE ( 'NONE', *, *, #29909, .F. ) ;
#46660=ORIENTED_EDGE ( 'NONE', *, *, #49148, .F. ) ;
#46676=ORIENTED_EDGE ( 'NONE', *, *, #82413, .F. ) ;
#46693=ORIENTED_EDGE ( 'NONE', *, *, #34285, .T. ) ;
#46855=DIRECTION ( 'NONE',  ( 0.000000000000000000, 6.982966722218760189E-15, -1.000000000000000000 ) ) ;
#46873=LINE ( 'NONE', #26018, #62359 ) ;
#46904=DIRECTION ( 'NONE',  ( -0.000000000000000000, 1.000000000000000000, -0.000000000000000000 ) ) ;
#46916=ORIENTED_EDGE ( 'NONE', *, *, #72739, .F. ) ;
#46917=ORIENTED_EDGE ( 'NONE', *, *, #59587, .T. ) ;
#46983=CARTESIAN_POINT ( 'NONE',  ( -215.9000000000000057, 104.7749999999999915, -41.27499999999999858 ) ) ;
#46988=ADVANCED_FACE ( 'NONE', ( #58812, #80187 ), #24320, .T. ) ;
#47019=ORIENTED_EDGE ( 'NONE', *, *, #69839, .F. ) ;
#47022=ORIENTED_EDGE ( 'NONE', *, *, #16649, .F. ) ;
#47054=CARTESIAN_POINT ( 'NONE',  ( -487.2989999999999782, 101.9113919710471947, 11.11250000000054072 ) ) ;
#47092=CARTESIAN_POINT ( 'NONE',  ( -492.0614999999999668, 93.66249999999999432, 11.11250000000040217 ) ) ;
#47107=DIRECTION ( 'NONE',  ( 1.000000000000000000, 0.000000000000000000, 0.000000000000000000 ) ) ;
#47151=VECTOR ( 'NONE', #76039, 1000.000000000000000 ) ;
#47167=DIRECTION ( 'NONE',  ( -1.000000000000000000, 0.000000000000000000, 0.000000000000000000 ) ) ;
#47182=DIRECTION ( 'NONE',  ( 1.000000000000000000, 0.000000000000000000, 0.000000000000000000 ) ) ;
#47206=ADVANCED_FACE ( 'NONE', ( #74871 ), #25824, .T. ) ;
#47227=LINE ( 'NONE', #74055, #8196 ) ;
#47251=DIRECTION ( 'NONE',  ( -1.000000000000000000, 0.000000000000000000, 0.000000000000000000 ) ) ;
#47264=AXIS2_PLACEMENT_3D ( 'NONE', #7359, #2792, #78212 ) ;
#47279=FACE_OUTER_BOUND ( 'NONE', #68106, .T. ) ;
#47281=LINE ( 'NONE', #83627, #49394 ) ;
#47322=ORIENTED_EDGE ( 'NONE', *, *, #29175, .T. ) ;
#47351=EDGE_LOOP ( 'NONE', ( #72871, #6332 ) ) ;
#47352=CARTESIAN_POINT ( 'NONE',  ( -487.2989999999999782, 100.8062500000000057, 86.36305401447658880 ) ) ;
#47386=( NAMED_UNIT ( * ) SI_UNIT ( $, .STERADIAN. ) SOLID_ANGLE_UNIT ( ) );
#47399=EDGE_CURVE ( 'NONE', #79779, #50718, #351, .T. ) ;
#47400=DIRECTION ( 'NONE',  ( 0.000000000000000000, 0.000000000000000000, -1.000000000000000000 ) ) ;
#47428=CARTESIAN_POINT ( 'NONE',  ( -47.15545942921612266, 92.90828646061743257, 75.16624513914106842 ) ) ;
#47434=ORIENTED_EDGE ( 'NONE', *, *, #19149, .T. ) ;
#47461=EDGE_LOOP ( 'NONE', ( #34298, #42411, #7249, #9814, #9752, #12603, #8664, #25088, #66014, #57791 ) ) ;
#47491=CARTESIAN_POINT ( 'NONE',  ( 0.000000000000000000, 93.07500000000001705, 0.000000000000000000 ) ) ;
#47499=DIRECTION ( 'NONE',  ( 0.000000000000000000, 0.000000000000000000, 1.000000000000000000 ) ) ;
#47505=DIRECTION ( 'NONE',  ( 0.000000000000000000, 0.000000000000000000, 1.000000000000000000 ) ) ;
#47514=ORIENTED_EDGE ( 'NONE', *, *, #3169, .T. ) ;
#47557=VERTEX_POINT ( 'NONE', #69464 ) ;
#47565=PLANE ( 'NONE',  #85179 ) ;
#47574=VECTOR ( 'NONE', #37697, 1000.000000000000000 ) ;
#47584=VECTOR ( 'NONE', #71516, 1000.000000000000000 ) ;
#47597=VECTOR ( 'NONE', #1854, 1000.000000000000114 ) ;
#47598=LINE ( 'NONE', #53953, #56367 ) ;
#47608=ADVANCED_FACE ( 'NONE', ( #76271, #11014, #80523 ), #14048, .F. ) ;
#47631=DIRECTION ( 'NONE',  ( 0.000000000000000000, 0.000000000000000000, 1.000000000000000000 ) ) ;
#47652=BREP_WITH_VOIDS ( 'NONE', #61879, ( #53332 ) );
#47677=ORIENTED_EDGE ( 'NONE', *, *, #83027, .F. ) ;
#47679=ORIENTED_EDGE ( 'NONE', *, *, #36211, .F. ) ;
#47684=CARTESIAN_POINT ( 'NONE',  ( -240.5296158183964792, 14.28750000000026077, 6.349999999999710099 ) ) ;
#47709=AXIS2_PLACEMENT_3D ( 'NONE', #76273, #36286, #57615 ) ;
#47721=ORIENTED_EDGE ( 'NONE', *, *, #6679, .F. ) ;
#47742=CARTESIAN_POINT ( 'NONE',  ( -4.442790029898877613, 70.75203571141577186, 118.2732005548771070 ) ) ;
#47751=CARTESIAN_POINT ( 'NONE',  ( 61.00843881761244347, 49.07499999999999574, -33.74458626278666884 ) ) ;
#47774=AXIS2_PLACEMENT_3D ( 'NONE', #19669, #12872, #67817 ) ;
#47782=LINE ( 'NONE', #11497, #11036 ) ;
#47792=CARTESIAN_POINT ( 'NONE',  ( -47.08824421440486674, 65.65858298468711496, 108.8036001757373299 ) ) ;
#47796=CARTESIAN_POINT ( 'NONE',  ( -9.196775925256822859, 91.17253193803733780, 117.9985040796144915 ) ) ;
#47825=LINE ( 'NONE', #49167, #3498 ) ;
#47844=DIRECTION ( 'NONE',  ( -0.2884130866282271777, 0.7071067811865476838, 0.6456143519637543848 ) ) ;
#47850=CARTESIAN_POINT ( 'NONE',  ( 0.000000000000000000, 93.07500000000001705, 0.000000000000000000 ) ) ;
#47852=DIRECTION ( 'NONE',  ( 0.000000000000000000, 0.5000000000000007772, -0.8660254037844381525 ) ) ;
#47865=VERTEX_POINT ( 'NONE', #17187 ) ;
#47871=DIRECTION ( 'NONE',  ( 0.000000000000000000, -0.4999999999999990563, -0.8660254037844392627 ) ) ;
#47878=VERTEX_POINT ( 'NONE', #39403 ) ;
#47879=ORIENTED_EDGE ( 'NONE', *, *, #12669, .F. ) ;
#47894=ORIENTED_EDGE ( 'NONE', *, *, #64470, .F. ) ;
#47921=ADVANCED_FACE ( 'NONE', ( #60282 ), #84851, .T. ) ;
#47928=DIRECTION ( 'NONE',  ( 1.000000000000000000, 0.000000000000000000, 0.000000000000000000 ) ) ;
#47934=ORIENTED_EDGE ( 'NONE', *, *, #64790, .T. ) ;
#47944=LINE ( 'NONE', #13454, #24456 ) ;
#47954=CARTESIAN_POINT ( 'NONE',  ( 0.000000000000000000, 92.07499999999998863, 0.000000000000000000 ) ) ;
#47971=CARTESIAN_POINT ( 'NONE',  ( -79.44498778673575146, 98.01532655701802810, 25.01765082793386696 ) ) ;
#47993=CARTESIAN_POINT ( 'NONE',  ( -41.60202597009397607, 40.59999999999997300, 50.85338361873603219 ) ) ;
#48032=EDGE_CURVE ( 'NONE', #11211, #1301, #61660, .T. ) ;
#48043=CARTESIAN_POINT ( 'NONE',  ( -446.0240000000000009, 53.97500000000000142, 50.79999999999999716 ) ) ;
#48067=EDGE_CURVE ( 'NONE', #8698, #21236, #33482, .T. ) ;
#48074=VECTOR ( 'NONE', #82749, 1000.000000000000000 ) ;
#48075=FACE_OUTER_BOUND ( 'NONE', #35808, .T. ) ;
#48076=PLANE ( 'NONE',  #27847 ) ;
#48082=LINE ( 'NONE', #34916, #43763 ) ;
#48101=FACE_OUTER_BOUND ( 'NONE', #83593, .T. ) ;
#48103=ORIENTED_EDGE ( 'NONE', *, *, #29175, .F. ) ;
#48105=CARTESIAN_POINT ( 'NONE',  ( -458.3598257906459708, 60.32499999999999574, -3.174999999999999822 ) ) ;
#48150=ORIENTED_EDGE ( 'NONE', *, *, #39639, .T. ) ;
#48168=EDGE_LOOP ( 'NONE', ( #28923, #77002 ) ) ;
#48187=AXIS2_PLACEMENT_3D ( 'NONE', #65750, #63988, #45301 ) ;
#48192=EDGE_CURVE ( 'NONE', #32697, #52469, #56147, .T. ) ;
#48258=EDGE_LOOP ( 'NONE', ( #74599, #46358, #61999, #15931 ) ) ;
#48269=AXIS2_PLACEMENT_3D ( 'NONE', #69430, #56678, #77143 ) ;
#48280=DIRECTION ( 'NONE',  ( 1.000000000000000000, 0.000000000000000000, 0.000000000000000000 ) ) ;
#48289=LINE ( 'NONE', #20621, #89273 ) ;
#48378=ADVANCED_FACE ( 'NONE', ( #23465 ), #66100, .F. ) ;
#48387=DIRECTION ( 'NONE',  ( 0.000000000000000000, 0.000000000000000000, -1.000000000000000000 ) ) ;
#48411=EDGE_CURVE ( 'NONE', #65784, #40115, #31581, .T. ) ;
#48413=ORIENTED_EDGE ( 'NONE', *, *, #62533, .F. ) ;
#48429=DIRECTION ( 'NONE',  ( -0.9130365726098601531, 0.000000000000000000, -0.4078776986755214828 ) ) ;
#48431=LINE ( 'NONE', #29379, #22347 ) ;
#48435=DIRECTION ( 'NONE',  ( -1.000000000000000000, 0.000000000000000000, 0.000000000000000000 ) ) ;
#48447=ADVANCED_FACE ( 'NONE', ( #11139 ), #38844, .T. ) ;
#48451=ORIENTED_EDGE ( 'NONE', *, *, #33785, .F. ) ;
#48463=ORIENTED_EDGE ( 'NONE', *, *, #73379, .F. ) ;
#48536=ADVANCED_FACE ( 'NONE', ( #34267 ), #82063, .T. ) ;
#48537=CARTESIAN_POINT ( 'NONE',  ( 50.30672865705777497, 91.74178678112681951, -72.48695520484585586 ) ) ;
#48544=DIRECTION ( 'NONE',  ( 0.000000000000000000, -0.8660254037844384856, 0.5000000000000003331 ) ) ;
#48549=VECTOR ( 'NONE', #68910, 1000.000000000000000 ) ;
#48551=AXIS2_PLACEMENT_3D ( 'NONE', #89060, #80023, #45455 ) ;
#48569=DIRECTION ( 'NONE',  ( 0.2645893543674792125, -0.6270931345857608807, -0.7326299707975406639 ) ) ;
#48593=CARTESIAN_POINT ( 'NONE',  ( 10.32955618830038347, 75.14983015127609178, 118.1053723791018086 ) ) ;
#48611=CARTESIAN_POINT ( 'NONE',  ( 4.665904304751416087E-15, 91.07499999999996021, -38.10000000000000142 ) ) ;
#48623=EDGE_CURVE ( 'NONE', #17788, #72087, #74776, .T. ) ;
#48670=CARTESIAN_POINT ( 'NONE',  ( -17.54031676229694270, 53.97499999999997300, 43.71138335376677020 ) ) ;
#48714=DIRECTION ( 'NONE',  ( 0.000000000000000000, -0.5000000000000007772, 0.8660254037844381525 ) ) ;
#48729=DIRECTION ( 'NONE',  ( -0.2884130866282260119, -0.7071067811865425767, 0.6456143519637603800 ) ) ;
#48741=EDGE_CURVE ( 'NONE', #10966, #3353, #11032, .T. ) ;
#48742=DIRECTION ( 'NONE',  ( -0.7071067811865475727, -0.7071067811865475727, -1.287852911526280419E-16 ) ) ;
#48779=CARTESIAN_POINT ( 'NONE',  ( -487.2989999999999782, 85.41360802895360393, 11.11250000000036131 ) ) ;
#48816=CIRCLE ( 'NONE', #15530, 11.17600000000001970 ) ;
#48833=CIRCLE ( 'NONE', #3922, 88.90000000000000568 ) ;
#48870=EDGE_CURVE ( 'NONE', #32697, #88397, #86024, .T. ) ;
#48908=ORIENTED_EDGE ( 'NONE', *, *, #27127, .T. ) ;
#48914=CARTESIAN_POINT ( 'NONE',  ( -492.0614999999999668, 14.28749999999982201, 90.48749999999999716 ) ) ;
#48928=ORIENTED_EDGE ( 'NONE', *, *, #64657, .T. ) ;
#48966=ORIENTED_EDGE ( 'NONE', *, *, #7024, .T. ) ;
#48970=ORIENTED_EDGE ( 'NONE', *, *, #43001, .F. ) ;
#48978=LINE ( 'NONE', #63530, #61292 ) ;
#48983=B_SPLINE_CURVE_WITH_KNOTS ( 'NONE', 3,
 ( #23278, #36439, #22815, #57760, #70054, #552, #1914, #85045, #50490, #43677, #9175, #36875, #64583, #50942, #78687, #51372, #37773, #31833, #72298, #4134, #45443, #59969, #30507, #30949, #32274 ),
 .UNSPECIFIED., .F., .F.,
 ( 4, 2, 2, 1, 2, 2, 2, 2, 2, 2, 2, 2, 4 ),
 ( 0.03942124974134118831, 0.04188566783051467235, 0.04311787687510139355, 0.04435008591968810782, 0.04558229496427482902, 0.04681450400886155022, 0.04927892209803499957, 0.05051113114262172077, 0.05174334018720844891, 0.05420775827638189825, 0.05543996732096862640, 0.05667217636555535454, 0.05913659445472881082 ),
 .UNSPECIFIED. ) ;
#48986=CARTESIAN_POINT ( 'NONE',  ( -446.0240000000000009, 53.97500000000000853, 101.5999999999999943 ) ) ;
#48993=DIRECTION ( 'NONE',  ( -0.1315836003796857501, 0.7863649282873461654, -0.6035859140758308428 ) ) ;
#49033=ORIENTED_EDGE ( 'NONE', *, *, #60031, .F. ) ;
#49044=CARTESIAN_POINT ( 'NONE',  ( -454.6936515812919879, 53.97500000000000142, 3.174999999999999822 ) ) ;
#49046=CARTESIAN_POINT ( 'NONE',  ( 4.867662263754145791, 70.79804876089910692, 118.4578822119320023 ) ) ;
#49069=ORIENTED_EDGE ( 'NONE', *, *, #67114, .T. ) ;
#49073=VECTOR ( 'NONE', #57262, 1000.000000000000000 ) ;
#49126=VECTOR ( 'NONE', #83290, 1000.000000000000000 ) ;
#49146=AXIS2_PLACEMENT_3D ( 'NONE', #65114, #58725, #85139 ) ;
#49148=EDGE_CURVE ( 'NONE', #41996, #26777, #76398, .T. ) ;
#49151=EDGE_CURVE ( 'NONE', #61703, #75492, #70946, .T. ) ;
#49167=CARTESIAN_POINT ( 'NONE',  ( -479.3614999999999782, 10.16305401447645984, 83.34375000000000000 ) ) ;
#49171=DIRECTION ( 'NONE',  ( -0.000000000000000000, 1.000000000000000000, -0.000000000000000000 ) ) ;
#49184=LINE ( 'NONE', #22407, #7079 ) ;
#49191=CARTESIAN_POINT ( 'NONE',  ( -15.89999999999999680, 53.97500000000000142, 50.79999999999999716 ) ) ;
#49218=DIRECTION ( 'NONE',  ( 0.000000000000000000, 0.000000000000000000, 1.000000000000000000 ) ) ;
#49225=EDGE_LOOP ( 'NONE', ( #81502, #75092, #47322, #61605, #36452 ) ) ;
#49258=ORIENTED_EDGE ( 'NONE', *, *, #63223, .F. ) ;
#49262=VECTOR ( 'NONE', #35581, 999.9999999999998863 ) ;
#49264=CARTESIAN_POINT ( 'NONE',  ( -487.2989999999999782, 14.28750000000026077, 15.87499999999969802 ) ) ;
#49268=CONICAL_SURFACE ( 'NONE', #60883, 89.90000000000000568, 0.7853981633974206344 ) ;
#49276=ADVANCED_FACE ( 'NONE', ( #77751, #27795 ), #41410, .T. ) ;
#49289=ORIENTED_EDGE ( 'NONE', *, *, #78891, .F. ) ;
#49300=LINE ( 'NONE', #63849, #23046 ) ;
#49304=DIRECTION ( 'NONE',  ( 0.000000000000000000, 0.000000000000000000, -1.000000000000000000 ) ) ;
#49305=VECTOR ( 'NONE', #63847, 999.9999999999998863 ) ;
#49364=ORIENTED_EDGE ( 'NONE', *, *, #70300, .T. ) ;
#49394=VECTOR ( 'NONE', #76803, 1000.000000000000000 ) ;
#49404=CARTESIAN_POINT ( 'NONE',  ( -487.2989999999999782, 86.51875000000001137, 94.61194598552339130 ) ) ;
#49425=AXIS2_PLACEMENT_3D ( 'NONE', #85956, #9195, #57774 ) ;
#49426=EDGE_LOOP ( 'NONE', ( #48966, #73392, #52999, #64831 ) ) ;
#49429=LINE ( 'NONE', #77165, #29324 ) ;
#49438=EDGE_LOOP ( 'NONE', ( #11631, #74495, #82946 ) ) ;
#49448=CARTESIAN_POINT ( 'NONE',  ( -76.47785380479396622, 54.92403073184157591, 30.82222824574506603 ) ) ;
#49454=CARTESIAN_POINT ( 'NONE',  ( -487.2989999999999782, 93.66249999999999432, 98.73639197104678544 ) ) ;
#49461=AXIS2_PLACEMENT_3D ( 'NONE', #9414, #64827, #52053 ) ;
#49509=CARTESIAN_POINT ( 'NONE',  ( 0.000000000000000000, 65.60000000000000853, -33.74458626278666884 ) ) ;
#49512=CARTESIAN_POINT ( 'NONE',  ( -465.6921742093550165, 47.62500000000000000, 3.174999999999999822 ) ) ;
#49538=DIRECTION ( 'NONE',  ( -0.5610517121635795190, -0.5610517121635953952, -0.6086394273760236118 ) ) ;
#49554=DIRECTION ( 'NONE',  ( 0.000000000000000000, 0.000000000000000000, 1.000000000000000000 ) ) ;
#49558=CARTESIAN_POINT ( 'NONE',  ( 0.000000000000000000, 91.07499999999996021, 0.000000000000000000 ) ) ;
#49575=CARTESIAN_POINT ( 'NONE',  ( 10.01853287408365745, 90.23518421848368121, 117.9321046141928662 ) ) ;
#49578=EDGE_LOOP ( 'NONE', ( #75764, #70168, #77251, #61527 ) ) ;
#49582=LINE ( 'NONE', #85039, #79507 ) ;
#49587=VERTEX_POINT ( 'NONE', #59950 ) ;
#49596=LINE ( 'NONE', #42775, #50061 ) ;
#49618=CARTESIAN_POINT ( 'NONE',  ( -41.60202597009397607, 40.59999999999997300, 54.55338361873603503 ) ) ;
#49635=LINE ( 'NONE', #36484, #70959 ) ;
#49639=AXIS2_PLACEMENT_3D ( 'NONE', #34534, #21365, #26819 ) ;
#49647=DIRECTION ( 'NONE',  ( -1.821299053822143307E-16, 0.000000000000000000, 1.000000000000000000 ) ) ;
#49706=ORIENTED_EDGE ( 'NONE', *, *, #17109, .F. ) ;
#49713=CARTESIAN_POINT ( 'NONE',  ( -34.53140813619931748, 54.97499999999996589, 35.02576496182814481 ) ) ;
#49735=CARTESIAN_POINT ( 'NONE',  ( -492.0614999999999668, 93.66249999999999432, 6.350000000000409983 ) ) ;
#49750=DIRECTION ( 'NONE',  ( 0.000000000000000000, 0.000000000000000000, 1.000000000000000000 ) ) ;
#49775=VERTEX_POINT ( 'NONE', #66114 ) ;
#49777=DIRECTION ( 'NONE',  ( 0.000000000000000000, 0.000000000000000000, 1.000000000000000000 ) ) ;
#49800=DIRECTION ( 'NONE',  ( 0.000000000000000000, 0.000000000000000000, 1.000000000000000000 ) ) ;
#49802=DIRECTION ( 'NONE',  ( 0.000000000000000000, -1.000000000000000000, 0.000000000000000000 ) ) ;
#49806=CARTESIAN_POINT ( 'NONE',  ( -55.59646339173026774, 54.92078272276780382, 70.77919445882530169 ) ) ;
#49900=EDGE_LOOP ( 'NONE', ( #42904, #36781, #16566, #14009, #16313 ) ) ;
#49919=CARTESIAN_POINT ( 'NONE',  ( -446.0240000000000009, 3.174999999999999822, -1.387778780781445991E-14 ) ) ;
#49941=VECTOR ( 'NONE', #20203, 1000.000000000000114 ) ;
#49956=DIRECTION ( 'NONE',  ( 1.000000000000000000, 0.000000000000000000, -0.000000000000000000 ) ) ;
#49982=CARTESIAN_POINT ( 'NONE',  ( -6.309812078926137602, 71.61276833203498882, 118.1896733548958451 ) ) ;
#49985=EDGE_CURVE ( 'NONE', #14599, #13052, #12963, .T. ) ;
#49994=DIRECTION ( 'NONE',  ( 0.000000000000000000, -0.5000000000000087708, 0.8660254037844336006 ) ) ;
#50003=ORIENTED_EDGE ( 'NONE', *, *, #25778, .F. ) ;
#50025=ORIENTED_EDGE ( 'NONE', *, *, #56028, .T. ) ;
#50031=EDGE_CURVE ( 'NONE', #72087, #17788, #74915, .T. ) ;
#50036=CARTESIAN_POINT ( 'NONE',  ( -0.8226739993993643640, 95.14999999999996305, 118.3559999999999519 ) ) ;
#50044=DIRECTION ( 'NONE',  ( 0.000000000000000000, 0.000000000000000000, -1.000000000000000000 ) ) ;
#50061=VECTOR ( 'NONE', #50044, 1000.000000000000000 ) ;
#50086=LINE ( 'NONE', #71012, #27824 ) ;
#50089=CARTESIAN_POINT ( 'NONE',  ( -487.2989999999999782, 100.8062500000000057, 94.61194598552329182 ) ) ;
#50099=FACE_OUTER_BOUND ( 'NONE', #84093, .T. ) ;
#50104=ORIENTED_EDGE ( 'NONE', *, *, #67059, .T. ) ;
#50120=ORIENTED_EDGE ( 'NONE', *, *, #10848, .F. ) ;
#50128=DIRECTION ( 'NONE',  ( -1.000000000000000000, 0.000000000000000000, 0.000000000000000000 ) ) ;
#50141=DIRECTION ( 'NONE',  ( 0.2130003897598659046, -0.000000000000000000, 0.9770521142508956647 ) ) ;
#50154=FACE_OUTER_BOUND ( 'NONE', #11655, .T. ) ;
#50180=CARTESIAN_POINT ( 'NONE',  ( 0.000000000000000000, 101.6000000000000227, 0.000000000000000000 ) ) ;
#50204=CARTESIAN_POINT ( 'NONE',  ( -50.35902679310718355, 64.60000000000000853, 27.95514712793348977 ) ) ;
#50244=DIRECTION ( 'NONE',  ( 0.000000000000000000, 0.000000000000000000, 1.000000000000000000 ) ) ;
#50248=ORIENTED_EDGE ( 'NONE', *, *, #54100, .F. ) ;
#50251=CARTESIAN_POINT ( 'NONE',  ( -55.95243198108136085, 55.97500000000000142, 70.69974874213239957 ) ) ;
#50305=ORIENTED_EDGE ( 'NONE', *, *, #19953, .T. ) ;
#50313=VERTEX_POINT ( 'NONE', #55487 ) ;
#50323=CIRCLE ( 'NONE', #64798, 88.90000000000000568 ) ;
#50339=CONICAL_SURFACE ( 'NONE', #16962, 39.10000000000005116, 0.7853981633974587151 ) ;
#50365=ORIENTED_EDGE ( 'NONE', *, *, #83685, .F. ) ;
#50367=ORIENTED_EDGE ( 'NONE', *, *, #34180, .F. ) ;
#50379=CARTESIAN_POINT ( 'NONE',  ( -487.2989999999999782, 14.28750000000026077, 6.349999999999710099 ) ) ;
#50400=CARTESIAN_POINT ( 'NONE',  ( 12.70000000000000107, 82.54999999999999716, 117.8738102209307641 ) ) ;
#50404=ORIENTED_EDGE ( 'NONE', *, *, #74595, .F. ) ;
#50437=CARTESIAN_POINT ( 'NONE',  ( -5.586631576746658112, 71.22609051415520298, 118.2265399586805472 ) ) ;
#50456=DIRECTION ( 'NONE',  ( -0.4634479843259246556, 0.000000000000000000, -0.8861241255175470455 ) ) ;
#50490=CARTESIAN_POINT ( 'NONE',  ( 10.91960523489288093, 76.24982137887049305, 117.8513599261979721 ) ) ;
#50510=ORIENTED_EDGE ( 'NONE', *, *, #76363, .F. ) ;
#50516=ORIENTED_EDGE ( 'NONE', *, *, #48870, .T. ) ;
#50522=LINE ( 'NONE', #43705, #35388 ) ;
#50540=DIRECTION ( 'NONE',  ( 1.000000000000000000, 0.000000000000000000, 0.000000000000000000 ) ) ;
#50553=CARTESIAN_POINT ( 'NONE',  ( -48.02966122971775320, 65.60000000000000853, -8.747637655308301746E-15 ) ) ;
#50592=VERTEX_POINT ( 'NONE', #68601 ) ;
#50603=DIRECTION ( 'NONE',  ( 0.000000000000000000, 0.000000000000000000, -1.000000000000000000 ) ) ;
#50607=ORIENTED_EDGE ( 'NONE', *, *, #60600, .T. ) ;
#50610=ORIENTED_EDGE ( 'NONE', *, *, #11656, .F. ) ;
#50636=FACE_OUTER_BOUND ( 'NONE', #12442, .T. ) ;
#50652=CYLINDRICAL_SURFACE ( 'NONE', #51096, 17.33514202138210081 ) ;
#50656=AXIS2_PLACEMENT_3D ( 'NONE', #89656, #19265, #5642 ) ;
#50681=ORIENTED_EDGE ( 'NONE', *, *, #65774, .F. ) ;
#50718=VERTEX_POINT ( 'NONE', #35853 ) ;
#50730=ORIENTED_EDGE ( 'NONE', *, *, #83685, .T. ) ;
#50747=VERTEX_POINT ( 'NONE', #49919 ) ;
#50759=CARTESIAN_POINT ( 'NONE',  ( -34.75390121890993811, 65.59999999999998010, 71.80362806563780964 ) ) ;
#50803=VECTOR ( 'NONE', #17036, 1000.000000000000000 ) ;
#50807=DIRECTION ( 'NONE',  ( 1.000000000000000000, 0.000000000000000000, 0.000000000000000000 ) ) ;
#50825=ORIENTED_EDGE ( 'NONE', *, *, #33334, .T. ) ;
#50865=FACE_OUTER_BOUND ( 'NONE', #24819, .T. ) ;
#50876=AXIS2_PLACEMENT_3D ( 'NONE', #56470, #22427, #43287 ) ;
#50882=DIRECTION ( 'NONE',  ( 0.9130365726098600421, 0.000000000000000000, 0.4078776986755216494 ) ) ;
#50928=ORIENTED_EDGE ( 'NONE', *, *, #53404, .T. ) ;
#50942=CARTESIAN_POINT ( 'NONE',  ( 8.316536451391945306, 73.07542579002461025, 118.0638868015453795 ) ) ;
#50954=AXIS2_PLACEMENT_3D ( 'NONE', #23907, #16639, #50244 ) ;
#50970=CARTESIAN_POINT ( 'NONE',  ( -479.3614999999999782, 7.143750000000339995, 6.988054014476269948 ) ) ;
#50972=ORIENTED_EDGE ( 'NONE', *, *, #983, .T. ) ;
#51001=CARTESIAN_POINT ( 'NONE',  ( -450.8499999999999659, 53.97500000000000142, -2.412999999999919876 ) ) ;
#51008=EDGE_CURVE ( 'NONE', #76709, #72100, #13083, .T. ) ;
#51041=ORIENTED_EDGE ( 'NONE', *, *, #26812, .T. ) ;
#51042=CIRCLE ( 'NONE', #29341, 4.762500000000002842 ) ;
#51060=CARTESIAN_POINT ( 'NONE',  ( -479.3614999999999782, 10.16305401447645984, 83.34375000000000000 ) ) ;
#51069=PLANE ( 'NONE',  #22684 ) ;
#51096=AXIS2_PLACEMENT_3D ( 'NONE', #57016, #28884, #49304 ) ;
#51098=CARTESIAN_POINT ( 'NONE',  ( -254.0000000000000000, 104.7749999999999915, 50.79999999999999716 ) ) ;
#51102=ORIENTED_EDGE ( 'NONE', *, *, #8054, .T. ) ;
#51133=VECTOR ( 'NONE', #72072, 1000.000000000000114 ) ;
#51171=VERTEX_POINT ( 'NONE', #5676 ) ;
#51254=ORIENTED_EDGE ( 'NONE', *, *, #71311, .F. ) ;
#51285=EDGE_CURVE ( 'NONE', #7646, #79779, #6123, .T. ) ;
#51290=EDGE_CURVE ( 'NONE', #80402, #87454, #67886, .T. ) ;
#51309=VERTEX_POINT ( 'NONE', #32911 ) ;
#51314=EDGE_CURVE ( 'NONE', #66470, #50313, #28608, .T. ) ;
#51315=EDGE_LOOP ( 'NONE', ( #36793, #68870, #4328, #9152 ) ) ;
#51341=DIRECTION ( 'NONE',  ( 1.000000000000000000, 0.000000000000000000, 0.000000000000000000 ) ) ;
#51360=ORIENTED_EDGE ( 'NONE', *, *, #43886, .T. ) ;
#51365=DIRECTION ( 'NONE',  ( 0.000000000000000000, 1.000000000000000000, 0.000000000000000000 ) ) ;
#51372=CARTESIAN_POINT ( 'NONE',  ( 7.341135922521115909, 72.30123413915578112, 118.1286081293353760 ) ) ;
#51377=VERTEX_POINT ( 'NONE', #69684 ) ;
#51415=VECTOR ( 'NONE', #10467, 1000.000000000000000 ) ;
#51418=VECTOR ( 'NONE', #54194, 1000.000000000000000 ) ;
#51425=DIRECTION ( 'NONE',  ( 0.000000000000000000, 0.000000000000000000, -1.000000000000000000 ) ) ;
#51429=CARTESIAN_POINT ( 'NONE',  ( -487.2989999999999782, 89.53805401447711176, 3.968750000000410338 ) ) ;
#51431=DIRECTION ( 'NONE',  ( 0.000000000000000000, -1.000000000000000000, -7.536132396315209176E-17 ) ) ;
#51436=CYLINDRICAL_SURFACE ( 'NONE', #71156, 4.762500000000002842 ) ;
#51442=ORIENTED_EDGE ( 'NONE', *, *, #74407, .F. ) ;
#51455=EDGE_CURVE ( 'NONE', #59609, #27384, #1986, .T. ) ;
#51476=DIRECTION ( 'NONE',  ( -1.000000000000000000, 0.000000000000000000, 0.000000000000000000 ) ) ;
#51501=FACE_BOUND ( 'NONE', #55218, .T. ) ;
#51554=VECTOR ( 'NONE', #23359, 1000.000000000000114 ) ;
#51579=CARTESIAN_POINT ( 'NONE',  ( -462.0260000000000105, 41.27499999999999858, 3.174999999999999822 ) ) ;
#51594=FACE_OUTER_BOUND ( 'NONE', #28245, .T. ) ;
#51599=ORIENTED_EDGE ( 'NONE', *, *, #48032, .F. ) ;
#51625=CARTESIAN_POINT ( 'NONE',  ( -254.0000000000000000, 104.7749999999999915, -41.27499999999999858 ) ) ;
#51727=ORIENTED_EDGE ( 'NONE', *, *, #82413, .T. ) ;
#51742=DIRECTION ( 'NONE',  ( 0.000000000000000000, -1.000000000000000000, 0.000000000000000000 ) ) ;
#51746=ORIENTED_EDGE ( 'NONE', *, *, #55610, .F. ) ;
#51757=CARTESIAN_POINT ( 'NONE',  ( -465.6921742093539933, 60.32499999999999574, 3.174999999999999822 ) ) ;
#51806=CARTESIAN_POINT ( 'NONE',  ( 7.730661649919364997, 92.63472181420671347, 118.3041290865632220 ) ) ;
#51831=ORIENTED_EDGE ( 'NONE', *, *, #76003, .T. ) ;
#51837=ORIENTED_EDGE ( 'NONE', *, *, #83008, .T. ) ;
#51905=CARTESIAN_POINT ( 'NONE',  ( -5.625308623692421683, 71.15616178428264504, 118.4230398497201122 ) ) ;
#51918=AXIS2_PLACEMENT_3D ( 'NONE', #43609, #52193, #73111 ) ;
#51935=CONICAL_SURFACE ( 'NONE', #73745, 88.90000000000000568, 0.7853981633974621568 ) ;
#51985=DIRECTION ( 'NONE',  ( 0.000000000000000000, 0.000000000000000000, 1.000000000000000000 ) ) ;
#51986=CARTESIAN_POINT ( 'NONE',  ( 0.000000000000000000, 65.60000000000000853, 0.000000000000000000 ) ) ;
#51997=AXIS2_PLACEMENT_3D ( 'NONE', #81001, #25556, #88258 ) ;
#52003=ADVANCED_FACE ( 'NONE', ( #85441 ), #57699, .F. ) ;
#52006=DIRECTION ( 'NONE',  ( 0.000000000000000000, -0.8660254037844427044, 0.4999999999999928391 ) ) ;
#52031=ORIENTED_EDGE ( 'NONE', *, *, #43886, .F. ) ;
#52044=VERTEX_POINT ( 'NONE', #17269 ) ;
#52053=DIRECTION ( 'NONE',  ( 0.000000000000000000, 0.000000000000000000, 1.000000000000000000 ) ) ;
#52070=CARTESIAN_POINT ( 'NONE',  ( -479.3614999999999782, 86.51875000000001137, 86.36305401447658880 ) ) ;
#52129=CARTESIAN_POINT ( 'NONE',  ( -487.2989999999999782, 14.28750000000023945, 19.36139197104649767 ) ) ;
#52182=CONICAL_SURFACE ( 'NONE', #34837, 16.33514202138213633, 0.7853981633974430610 ) ;
#52193=DIRECTION ( 'NONE',  ( 0.000000000000000000, 1.809101308280369915E-15, -1.000000000000000000 ) ) ;
#52243=CARTESIAN_POINT ( 'NONE',  ( 1.664568416404320850, 95.16759698565884662, 118.5470925690480755 ) ) ;
#52295=DIRECTION ( 'NONE',  ( 0.000000000000000000, 0.000000000000000000, -1.000000000000000000 ) ) ;
#52334=CARTESIAN_POINT ( 'NONE',  ( -458.3598257906459708, 47.62500000000000000, 3.174999999999999822 ) ) ;
#52337=DIRECTION ( 'NONE',  ( 0.000000000000000000, -0.000000000000000000, -1.000000000000000000 ) ) ;
#52359=EDGE_LOOP ( 'NONE', ( #33948, #62437, #67438, #6478, #77647 ) ) ;
#52386=CARTESIAN_POINT ( 'NONE',  ( -487.2989999999999782, 86.51875000000001137, 86.36305401447658880 ) ) ;
#52427=ADVANCED_FACE ( 'NONE', ( #80731 ), #67659, .T. ) ;
#52469=VERTEX_POINT ( 'NONE', #73448 ) ;
#52503=ORIENTED_EDGE ( 'NONE', *, *, #14953, .T. ) ;
#52518=ADVANCED_FACE ( 'NONE', ( #75703 ), #7558, .F. ) ;
#52534=VERTEX_POINT ( 'NONE', #13033 ) ;
#52571=CARTESIAN_POINT ( 'NONE',  ( -215.9000000000000057, 53.97500000000000142, 70.79999999999999716 ) ) ;
#52572=CARTESIAN_POINT ( 'NONE',  ( -12.37528545905534649, 85.43392152113592886, 117.9083718356618817 ) ) ;
#52595=ORIENTED_EDGE ( 'NONE', *, *, #73105, .T. ) ;
#52631=ADVANCED_FACE ( 'NONE', ( #71583 ), #65198, .T. ) ;
#52680=ORIENTED_EDGE ( 'NONE', *, *, #17514, .T. ) ;
#52682=CARTESIAN_POINT ( 'NONE',  ( 9.562607838165547491, 90.94827852097223797, 118.1711730385347607 ) ) ;
#52754=CARTESIAN_POINT ( 'NONE',  ( -254.0000000000000000, 3.174999999999999822, -41.27499999999999858 ) ) ;
#52757=CARTESIAN_POINT ( 'NONE',  ( -34.75390121890993100, 53.97499999999997300, 71.80362806563778122 ) ) ;
#52845=CARTESIAN_POINT ( 'NONE',  ( -48.02966122971777452, 100.5999999999999659, 106.4272185163641780 ) ) ;
#52855=CARTESIAN_POINT ( 'NONE',  ( -47.18030668273772221, 93.07500000000001705, 75.34738655934135920 ) ) ;
#52857=PLANE ( 'NONE',  #75712 ) ;
#52876=DIRECTION ( 'NONE',  ( 0.000000000000000000, 0.000000000000000000, 1.000000000000000000 ) ) ;
#52880=CIRCLE ( 'NONE', #48551, 118.5560000000000116 ) ;
#52905=PLANE ( 'NONE',  #4287 ) ;
#52949=DIRECTION ( 'NONE',  ( -0.000000000000000000, 1.000000000000000000, -0.000000000000000000 ) ) ;
#52983=CARTESIAN_POINT ( 'NONE',  ( -492.0614999999999668, 93.66249999999999432, 90.48749999999999716 ) ) ;
#52999=ORIENTED_EDGE ( 'NONE', *, *, #37668, .T. ) ;
#53010=DIRECTION ( 'NONE',  ( 0.000000000000000000, 0.000000000000000000, -1.000000000000000000 ) ) ;
#53045=VERTEX_POINT ( 'NONE', #68328 ) ;
#53055=CARTESIAN_POINT ( 'NONE',  ( -479.3614999999999782, 85.41360802895360393, 11.11250000000036131 ) ) ;
#53086=VERTEX_POINT ( 'NONE', #1867 ) ;
#53109=ORIENTED_EDGE ( 'NONE', *, *, #3146, .F. ) ;
#53141=AXIS2_PLACEMENT_3D ( 'NONE', #50204, #37485, #36144 ) ;
#53146=ORIENTED_EDGE ( 'NONE', *, *, #17093, .F. ) ;
#53160=CARTESIAN_POINT ( 'NONE',  ( 0.000000000000000000, 65.60000000000000853, 0.000000000000000000 ) ) ;
#53164=FACE_OUTER_BOUND ( 'NONE', #24586, .T. ) ;
#53197=EDGE_CURVE ( 'NONE', #59106, #50747, #66301, .T. ) ;
#53232=LINE ( 'NONE', #18748, #24631 ) ;
#53235=CARTESIAN_POINT ( 'NONE',  ( 0.000000000000000000, 65.60000000000000853, 0.000000000000000000 ) ) ;
#53242=EDGE_LOOP ( 'NONE', ( #77332, #51837, #43355, #12776, #37075 ) ) ;
#53253=CARTESIAN_POINT ( 'NONE',  ( -12.27767284950918203, 85.41138372342587104, 117.7174922484384467 ) ) ;
#53259=DIRECTION ( 'NONE',  ( 0.000000000000000000, 0.000000000000000000, -1.000000000000000000 ) ) ;
#53294=ORIENTED_EDGE ( 'NONE', *, *, #35821, .F. ) ;
#53308=CYLINDRICAL_SURFACE ( 'NONE', #41958, 4.762500000000000178 ) ;
#53328=CARTESIAN_POINT ( 'NONE',  ( -465.6921742093539933, 60.32499999999999574, 3.174999999999999822 ) ) ;
#53332=ORIENTED_CLOSED_SHELL ( 'NONE', *, #27142, .F. );
#53347=ADVANCED_FACE ( 'NONE', ( #88118, #12705 ), #87660, .T. ) ;
#53363=CARTESIAN_POINT ( 'NONE',  ( -48.26476610531311451, 53.97499999999997300, 65.76796570303405076 ) ) ;
#53404=EDGE_CURVE ( 'NONE', #35189, #40115, #10170, .T. ) ;
#53431=ORIENTED_EDGE ( 'NONE', *, *, #28757, .T. ) ;
#53473=ORIENTED_EDGE ( 'NONE', *, *, #70745, .T. ) ;
#53486=LINE ( 'NONE', #74415, #64277 ) ;
#53487=ORIENTED_EDGE ( 'NONE', *, *, #35928, .F. ) ;
#53529=DIRECTION ( 'NONE',  ( 1.000000000000000000, -7.570719237730591757E-15, 0.000000000000000000 ) ) ;
#53571=AXIS2_PLACEMENT_3D ( 'NONE', #86033, #37417, #78775 ) ;
#53580=CARTESIAN_POINT ( 'NONE',  ( 69.63919639214307722, 92.07499999999998863, -53.63573739454432854 ) ) ;
#53581=VERTEX_POINT ( 'NONE', #10788 ) ;
#53600=CYLINDRICAL_SURFACE ( 'NONE', #7632, 50.79999999999999716 ) ;
#53605=CARTESIAN_POINT ( 'NONE',  ( -487.2989999999999782, 21.43125000000035030, 6.988054014476359654 ) ) ;
#53648=EDGE_CURVE ( 'NONE', #65744, #53086, #44405, .T. ) ;
#53657=CARTESIAN_POINT ( 'NONE',  ( -215.9000000000000057, 53.97500000000000142, 30.79999999999999361 ) ) ;
#53666=DIRECTION ( 'NONE',  ( 0.000000000000000000, -1.000000000000000000, -6.982966722218760189E-15 ) ) ;
#53704=CARTESIAN_POINT ( 'NONE',  ( -10.93444747363166769, 88.86474737026325954, 117.8507171435055483 ) ) ;
#53711=LINE ( 'NONE', #59204, #16522 ) ;
#53751=CARTESIAN_POINT ( 'NONE',  ( -34.53140813619931748, 64.60000000000000853, 35.02576496182815191 ) ) ;
#53776=VERTEX_POINT ( 'NONE', #39393 ) ;
#53797=CARTESIAN_POINT ( 'NONE',  ( -57.68704571023340577, 88.97500000000002274, 67.38312395177700864 ) ) ;
#53803=VERTEX_POINT ( 'NONE', #20312 ) ;
#53861=VECTOR ( 'NONE', #16367, 1000.000000000000000 ) ;
#53883=ORIENTED_EDGE ( 'NONE', *, *, #11342, .T. ) ;
#53886=VECTOR ( 'NONE', #27991, 1000.000000000000114 ) ;
#53923=ORIENTED_EDGE ( 'NONE', *, *, #37728, .T. ) ;
#53950=DIRECTION ( 'NONE',  ( 1.000000000000000000, 0.000000000000000000, 0.000000000000000000 ) ) ;
#53952=CARTESIAN_POINT ( 'NONE',  ( -254.0000000000000000, 53.97500000000000142, 50.79999999999999716 ) ) ;
#53953=CARTESIAN_POINT ( 'NONE',  ( -240.5296158183964792, 93.66249999999999432, 85.72499999999999432 ) ) ;
#53961=B_SPLINE_CURVE_WITH_KNOTS ( 'NONE', 3,
 ( #62193, #48537, #69019, #70819 ),
 .UNSPECIFIED., .F., .F.,
 ( 4, 4 ),
 ( 0.000000000000000000, 0.001493295663798172414 ),
 .UNSPECIFIED. ) ;
#54038=DIRECTION ( 'NONE',  ( 8.659560562355022838E-17, 0.7071067811865401342, -0.7071067811865549002 ) ) ;
#54085=CARTESIAN_POINT ( 'NONE',  ( -30.86579703273523734, 65.59999999999998010, 73.54054752236282866 ) ) ;
#54088=VECTOR ( 'NONE', #55722, 1000.000000000000000 ) ;
#54090=EDGE_LOOP ( 'NONE', ( #40636, #50972, #62835, #38712 ) ) ;
#54100=EDGE_CURVE ( 'NONE', #53086, #55800, #23457, .T. ) ;
#54103=VERTEX_POINT ( 'NONE', #37516 ) ;
#54192=SURFACE_STYLE_USAGE ( .BOTH. , #26519 ) ;
#54194=DIRECTION ( 'NONE',  ( -1.821299053822143307E-16, 0.000000000000000000, 1.000000000000000000 ) ) ;
#54198=LINE ( 'NONE', #53751, #74386 ) ;
#54230=ORIENTED_EDGE ( 'NONE', *, *, #64663, .F. ) ;
#54245=ORIENTED_EDGE ( 'NONE', *, *, #31735, .T. ) ;
#54250=CARTESIAN_POINT ( 'NONE',  ( -12.60000000000000142, 82.54999999999999716, 117.6834004267381744 ) ) ;
#54312=DIRECTION ( 'NONE',  ( -1.821299053822143307E-16, 0.000000000000000000, 1.000000000000000000 ) ) ;
#54324=DIRECTION ( 'NONE',  ( -1.000000000000000000, -0.000000000000000000, -0.000000000000000000 ) ) ;
#54351=CARTESIAN_POINT ( 'NONE',  ( -12.70000000000000107, 82.54999999999999716, 117.8738102209307641 ) ) ;
#54355=CYLINDRICAL_SURFACE ( 'NONE', #24347, 12.70000000000000107 ) ;
#54396=CARTESIAN_POINT ( 'NONE',  ( 0.000000000000000000, 82.54999999999999716, 92.46299999999996544 ) ) ;
#54401=VECTOR ( 'NONE', #88241, 1000.000000000000114 ) ;
#54430=ORIENTED_EDGE ( 'NONE', *, *, #17403, .F. ) ;
#54435=VERTEX_POINT ( 'NONE', #35145 ) ;
#54442=CARTESIAN_POINT ( 'NONE',  ( 50.24780502318014896, 92.07499999999998863, -72.12189744004568581 ) ) ;
#54451=CIRCLE ( 'NONE', #15333, 17.33514202138209370 ) ;
#54511=CIRCLE ( 'NONE', #29923, 38.10000000000000853 ) ;
#54525=ORIENTED_EDGE ( 'NONE', *, *, #33688, .T. ) ;
#54543=CARTESIAN_POINT ( 'NONE',  ( -3.258242219038141485, 70.37154502160744585, 118.3118053218331767 ) ) ;
#54577=CIRCLE ( 'NONE', #87940, 16.33514202138210791 ) ;
#54610=B_SPLINE_CURVE_WITH_KNOTS ( 'NONE', 3,
 ( #73950, #31711, #66680, #52572, #45324, #60753, #73043, #11727, #38521, #32155, #5359, #66221, #4010, #26244, #45766, #81237, #88488, #4464, #59849, #25797, #59408, #87582, #39423, #67128, #87140 ),
 .UNSPECIFIED., .F., .F.,
 ( 4, 2, 2, 1, 2, 2, 2, 2, 2, 2, 2, 2, 4 ),
 ( 0.03973447012869897599, 0.04221846688269337983, 0.04346046525969059909, 0.04470246363668782530, 0.04594446201368504457, 0.04718646039068226383, 0.04967045714467674400, 0.05091245552167399102, 0.05215445389867124498, 0.05463845065266575290, 0.05588044902966299993, 0.05712244740666024001, 0.05960644416065473405 ),
 .UNSPECIFIED. ) ;
#54676=CARTESIAN_POINT ( 'NONE',  ( -47.13037117915683893, 92.74157015026722206, 74.98513935456327317 ) ) ;
#54703=AXIS2_PLACEMENT_3D ( 'NONE', #9934, #1781, #44423 ) ;
#54704=PLANE ( 'NONE',  #33712 ) ;
#54753=DIRECTION ( 'NONE',  ( -0.000000000000000000, 1.000000000000000000, -0.000000000000000000 ) ) ;
#54755=DIRECTION ( 'NONE',  ( -1.000000000000000000, 0.000000000000000000, 0.000000000000000000 ) ) ;
#54772=CARTESIAN_POINT ( 'NONE',  ( -254.0000000000000000, 3.174999999999999822, -41.27499999999999858 ) ) ;
#54774=FACE_OUTER_BOUND ( 'NONE', #82226, .T. ) ;
#54799=CIRCLE ( 'NONE', #56231, 3.700000000000001954 ) ;
#54822=EDGE_LOOP ( 'NONE', ( #71558, #89746, #41202 ) ) ;
#54825=CARTESIAN_POINT ( 'NONE',  ( -47.02966122971777452, 101.5999999999999943, 107.7386843274874053 ) ) ;
#54836=AXIS2_PLACEMENT_3D ( 'NONE', #15195, #50141, #57412 ) ;
#54850=LINE ( 'NONE', #41676, #8550 ) ;
#54851=ORIENTED_EDGE ( 'NONE', *, *, #73105, .F. ) ;
#54883=ORIENTED_EDGE ( 'NONE', *, *, #3639, .T. ) ;
#54899=EDGE_LOOP ( 'NONE', ( #61212, #63604 ) ) ;
#54914=DIRECTION ( 'NONE',  ( 0.4999999999999915623, -0.8660254037844433705, 0.000000000000000000 ) ) ;
#54941=ADVANCED_FACE ( 'NONE', ( #7792 ), #40958, .T. ) ;
#54991=DIRECTION ( 'NONE',  ( 0.000000000000000000, 0.000000000000000000, 1.000000000000000000 ) ) ;
#55037=ORIENTED_EDGE ( 'NONE', *, *, #64656, .T. ) ;
#55043=CARTESIAN_POINT ( 'NONE',  ( -47.05895527891580343, 65.62929404919808007, 108.8162712210547056 ) ) ;
#55073=DIRECTION ( 'NONE',  ( -0.4999999999999941158, 0.8660254037844420383, 0.000000000000000000 ) ) ;
#55086=SURFACE_STYLE_FILL_AREA ( #33778 ) ;
#55089=LINE ( 'NONE', #76013, #23904 ) ;
#55103=ORIENTED_EDGE ( 'NONE', *, *, #87131, .T. ) ;
#55119=LINE ( 'NONE', #1544, #79096 ) ;
#55169=EDGE_CURVE ( 'NONE', #78995, #4807, #60285, .T. ) ;
#55183=DIRECTION ( 'NONE',  ( -1.000000000000000000, 0.000000000000000000, 0.000000000000000000 ) ) ;
#55218=EDGE_LOOP ( 'NONE', ( #83365, #87719 ) ) ;
#55233=VECTOR ( 'NONE', #89304, 1000.000000000000000 ) ;
#55256=DIRECTION ( 'NONE',  ( 1.000000000000000000, 0.000000000000000000, 0.000000000000000000 ) ) ;
#55266=VECTOR ( 'NONE', #59539, 1000.000000000000000 ) ;
#55268=DIRECTION ( 'NONE',  ( 1.000000000000000000, 0.000000000000000000, 0.000000000000000000 ) ) ;
#55270=ORIENTED_EDGE ( 'NONE', *, *, #64204, .F. ) ;
#55283=CARTESIAN_POINT ( 'NONE',  ( -41.60202597009397607, 65.59999999999998010, 34.51824159735389230 ) ) ;
#55290=CARTESIAN_POINT ( 'NONE',  ( -465.6921742093539933, 60.32499999999999574, -3.174999999999999822 ) ) ;
#55322=DIRECTION ( 'NONE',  ( 0.000000000000000000, -3.491483361109380094E-15, 1.000000000000000000 ) ) ;
#55325=DIRECTION ( 'NONE',  ( 0.000000000000000000, 0.000000000000000000, 1.000000000000000000 ) ) ;
#55345=EDGE_CURVE ( 'NONE', #18243, #39332, #48431, .T. ) ;
#55346=CARTESIAN_POINT ( 'NONE',  ( -240.5296158183964792, 93.66249999999999432, 6.350000000000409983 ) ) ;
#55363=DIRECTION ( 'NONE',  ( 1.000000000000000000, 0.000000000000000000, 0.000000000000000000 ) ) ;
#55378=VERTEX_POINT ( 'NONE', #3447 ) ;
#55385=AXIS2_PLACEMENT_3D ( 'NONE', #63514, #84878, #9452 ) ;
#55389=ORIENTED_EDGE ( 'NONE', *, *, #72659, .F. ) ;
#55399=EDGE_LOOP ( 'NONE', ( #47934, #51254, #62242, #82391 ) ) ;
#55411=EDGE_CURVE ( 'NONE', #75550, #79764, #12161, .T. ) ;
#55423=ADVANCED_FACE ( 'NONE', ( #10694 ), #86149, .T. ) ;
#55437=DIRECTION ( 'NONE',  ( 0.000000000000000000, -0.5000000000000087708, 0.8660254037844336006 ) ) ;
#55438=ORIENTED_EDGE ( 'NONE', *, *, #33164, .F. ) ;
#55452=CARTESIAN_POINT ( 'NONE',  ( -487.2989999999999782, 18.41194598552320016, 97.63125000000000853 ) ) ;
#55478=AXIS2_PLACEMENT_3D ( 'NONE', #71013, #8329, #36487 ) ;
#55487=CARTESIAN_POINT ( 'NONE',  ( -472.4400000000000546, 53.97500000000000142, -3.174999999999999822 ) ) ;
#55498=EDGE_CURVE ( 'NONE', #2162, #1004, #23020, .T. ) ;
#55514=ORIENTED_EDGE ( 'NONE', *, *, #1403, .T. ) ;
#55523=VERTEX_POINT ( 'NONE', #83277 ) ;
#55540=CONICAL_SURFACE ( 'NONE', #43765, 10.41399999999997839, 0.7853981633974744803 ) ;
#55544=CYLINDRICAL_SURFACE ( 'NONE', #73872, 20.00000000000000355 ) ;
#55547=FACE_OUTER_BOUND ( 'NONE', #66934, .T. ) ;
#55560=DIRECTION ( 'NONE',  ( 0.000000000000000000, 1.000000000000000000, 0.000000000000000000 ) ) ;
#55596=LINE ( 'NONE', #1577, #20684 ) ;
#55610=EDGE_CURVE ( 'NONE', #56124, #53803, #14235, .T. ) ;
#55628=EDGE_CURVE ( 'NONE', #87146, #16628, #20847, .T. ) ;
#55683=ADVANCED_FACE ( 'NONE', ( #61584 ), #75239, .T. ) ;
#55722=DIRECTION ( 'NONE',  ( 0.000000000000000000, -1.682382052829014912E-15, -1.000000000000000000 ) ) ;
#55735=DIRECTION ( 'NONE',  ( 0.000000000000000000, 0.000000000000000000, -1.000000000000000000 ) ) ;
#55745=COLOUR_RGB ( '', 0.31764706, 0.68627451, 0.89019608) ;
#55763=CARTESIAN_POINT ( 'NONE',  ( 0.000000000000000000, 93.07500000000001705, 0.000000000000000000 ) ) ;
#55770=DIRECTION ( 'NONE',  ( 0.000000000000000000, 1.000000000000000000, 0.000000000000000000 ) ) ;
#55800=VERTEX_POINT ( 'NONE', #1633 ) ;
#55802=ADVANCED_FACE ( 'NONE', ( #1175 ), #28157, .T. ) ;
#55855=CARTESIAN_POINT ( 'NONE',  ( 4.087783556564577481, 70.51867047662535981, 118.4861746650021104 ) ) ;
#55859=VERTEX_POINT ( 'NONE', #30222 ) ;
#55861=CARTESIAN_POINT ( 'NONE',  ( -446.0240000000000009, 93.66249999999999432, 11.11250000000040217 ) ) ;
#55863=AXIS2_PLACEMENT_3D ( 'NONE', #21062, #29664, #21521 ) ;
#55879=CARTESIAN_POINT ( 'NONE',  ( -46.60773131249376888, 65.60000000000000853, -44.42500552774628630 ) ) ;
#55884=AXIS2_PLACEMENT_3D ( 'NONE', #68800, #27455, #18858 ) ;
#55934=DIRECTION ( 'NONE',  ( 1.000000000000000000, 0.000000000000000000, 0.000000000000000000 ) ) ;
#55937=CARTESIAN_POINT ( 'NONE',  ( 0.8234126494891776948, 95.12992737732547255, 118.3538578355079522 ) ) ;
#55952=ORIENTED_EDGE ( 'NONE', *, *, #82525, .T. ) ;
#55956=DIRECTION ( 'NONE',  ( 0.000000000000000000, 5.300584669389750404E-15, -1.000000000000000000 ) ) ;
#55998=DIRECTION ( 'NONE',  ( -1.000000000000000000, -0.000000000000000000, -0.000000000000000000 ) ) ;
#56007=LINE ( 'NONE', #70570, #49262 ) ;
#56017=EDGE_CURVE ( 'NONE', #55800, #46111, #16591, .T. ) ;
#56025=DIRECTION ( 'NONE',  ( 0.000000000000000000, 0.000000000000000000, -1.000000000000000000 ) ) ;
#56026=CARTESIAN_POINT ( 'NONE',  ( -254.0000000000000000, 14.28749999999982201, 90.48749999999999716 ) ) ;
#56028=EDGE_CURVE ( 'NONE', #55859, #14474, #72007, .T. ) ;
#56040=CIRCLE ( 'NONE', #70533, 117.5559999999999974 ) ;
#56044=CARTESIAN_POINT ( 'NONE',  ( -487.2989999999999782, 6.038608028953049711, 90.48749999999999716 ) ) ;
#56052=CARTESIAN_POINT ( 'NONE',  ( -492.0614999999999668, 93.66249999999999432, 15.87500000000039968 ) ) ;
#56106=FACE_OUTER_BOUND ( 'NONE', #79916, .T. ) ;
#56108=DIRECTION ( 'NONE',  ( -6.245004513516504751E-15, 0.000000000000000000, -1.000000000000000000 ) ) ;
#56124=VERTEX_POINT ( 'NONE', #19707 ) ;
#56147=LINE ( 'NONE', #70253, #42787 ) ;
#56164=AXIS2_PLACEMENT_3D ( 'NONE', #8537, #77130, #29879 ) ;
#56176=DIRECTION ( 'NONE',  ( 0.000000000000000000, -0.000000000000000000, -1.000000000000000000 ) ) ;
#56192=PLANE ( 'NONE',  #61086 ) ;
#56215=LINE ( 'NONE', #37149, #16615 ) ;
#56231=AXIS2_PLACEMENT_3D ( 'NONE', #89365, #75728, #88472 ) ;
#56251=CARTESIAN_POINT ( 'NONE',  ( -48.26476610531312872, 65.59999999999998010, 65.76796570303407918 ) ) ;
#56254=LINE ( 'NONE', #14961, #57393 ) ;
#56309=CARTESIAN_POINT ( 'NONE',  ( 11.41159535906576217, 76.91451165865561279, 118.0059465515839747 ) ) ;
#56343=VECTOR ( 'NONE', #74620, 1000.000000000000000 ) ;
#56361=DIRECTION ( 'NONE',  ( 0.000000000000000000, 0.000000000000000000, 1.000000000000000000 ) ) ;
#56367=VECTOR ( 'NONE', #88961, 1000.000000000000000 ) ;
#56386=DIRECTION ( 'NONE',  ( 0.000000000000000000, 0.8660254037844428154, -0.4999999999999928946 ) ) ;
#56397=VECTOR ( 'NONE', #80165, 1000.000000000000000 ) ;
#56406=CARTESIAN_POINT ( 'NONE',  ( -1.790903581468949841E-22, 95.14999999999999147, 118.3560000000000088 ) ) ;
#56428=EDGE_CURVE ( 'NONE', #18305, #63160, #85093, .T. ) ;
#56470=CARTESIAN_POINT ( 'NONE',  ( -64.50026246089650783, 64.60000000000000853, 59.61038444174924678 ) ) ;
#56475=CARTESIAN_POINT ( 'NONE',  ( -487.2989999999999782, 89.53805401447711176, 3.968750000000410338 ) ) ;
#56505=CARTESIAN_POINT ( 'NONE',  ( -40.89999999999999858, 53.97500000000000142, 70.79999999999999716 ) ) ;
#56518=CARTESIAN_POINT ( 'NONE',  ( -254.0000000000000000, 93.66249999999999432, 90.48749999999999716 ) ) ;
#56524=CARTESIAN_POINT ( 'NONE',  ( -546.0365000000000464, 53.97500000000000142, 50.79999999999999716 ) ) ;
#56540=ORIENTED_EDGE ( 'NONE', *, *, #72739, .T. ) ;
#56559=AXIS2_PLACEMENT_3D ( 'NONE', #63137, #84046, #42671 ) ;
#56604=ADVANCED_FACE ( 'NONE', ( #67295 ), #19163, .T. ) ;
#56616=AXIS2_PLACEMENT_3D ( 'NONE', #38662, #66362, #87276 ) ;
#56618=CARTESIAN_POINT ( 'NONE',  ( -24.20305689751608824, 53.97499999999997300, 58.62596543806478877 ) ) ;
#56620=CARTESIAN_POINT ( 'NONE',  ( -12.67976079355167052, 81.71985538306350350, 117.8759963413547212 ) ) ;
#56637=AXIS2_PLACEMENT_3D ( 'NONE', #56518, #36090, #63346 ) ;
#56662=ORIENTED_EDGE ( 'NONE', *, *, #15878, .T. ) ;
#56676=EDGE_LOOP ( 'NONE', ( #72423, #7837, #23913, #4155 ) ) ;
#56678=DIRECTION ( 'NONE',  ( -0.000000000000000000, 1.000000000000000000, 0.000000000000000000 ) ) ;
#56680=FACE_OUTER_BOUND ( 'NONE', #66299, .T. ) ;
#56709=VERTEX_POINT ( 'NONE', #56800 ) ;
#56710=VERTEX_POINT ( 'NONE', #20951 ) ;
#56774=CARTESIAN_POINT ( 'NONE',  ( -30.89999999999999858, 53.97500000000000142, 50.79999999999999716 ) ) ;
#56780=CARTESIAN_POINT ( 'NONE',  ( -74.56320856954198462, 53.97500000000000142, 30.79999999999999361 ) ) ;
#56787=ADVANCED_FACE ( 'NONE', ( #4427 ), #87541, .F. ) ;
#56800=CARTESIAN_POINT ( 'NONE',  ( -479.3614999999999782, 14.28750000000036025, 2.863608028952929985 ) ) ;
#56811=LINE ( 'NONE', #8696, #16133 ) ;
#56812=ORIENTED_EDGE ( 'NONE', *, *, #35756, .T. ) ;
#56830=AXIS2_PLACEMENT_3D ( 'NONE', #24282, #37460, #73303 ) ;
#56842=CARTESIAN_POINT ( 'NONE',  ( 10.70251037890477797, 89.21217201404442676, 117.8713340830158955 ) ) ;
#56850=LINE ( 'NONE', #62774, #67875 ) ;
#56860=EDGE_CURVE ( 'NONE', #1971, #38989, #32554, .T. ) ;
#56875=ORIENTED_EDGE ( 'NONE', *, *, #76242, .F. ) ;
#56878=ORIENTED_EDGE ( 'NONE', *, *, #63650, .T. ) ;
#56936=DIRECTION ( 'NONE',  ( -1.000000000000000000, 0.000000000000000000, 0.000000000000000000 ) ) ;
#56947=PLANE ( 'NONE',  #4275 ) ;
#56974=ORIENTED_EDGE ( 'NONE', *, *, #25265, .F. ) ;
#57016=CARTESIAN_POINT ( 'NONE',  ( -41.60202597009397607, 65.59999999999998010, 50.85338361873603219 ) ) ;
#57068=CARTESIAN_POINT ( 'NONE',  ( -54.98109326260873786, 54.34217962558955861, 70.79744912815033331 ) ) ;
#57084=AXIS2_PLACEMENT_3D ( 'NONE', #22484, #46904, #80128 ) ;
#57096=CARTESIAN_POINT ( 'NONE',  ( -487.2989999999999782, 86.51875000000001137, 86.36305401447658880 ) ) ;
#57111=DIRECTION ( 'NONE',  ( -0.000000000000000000, -1.000000000000000000, 0.000000000000000000 ) ) ;
#57117=ORIENTED_EDGE ( 'NONE', *, *, #27037, .F. ) ;
#57140=ORIENTED_EDGE ( 'NONE', *, *, #14847, .F. ) ;
#57145=PRODUCT_DEFINITION ( 'UNKNOWN', '', #5804, #62612 ) ;
#57153=FILL_AREA_STYLE_COLOUR ( '', #55745 ) ;
#57205=FACE_BOUND ( 'NONE', #35800, .T. ) ;
#57206=DIRECTION ( 'NONE',  ( 0.000000000000000000, 0.000000000000000000, 1.000000000000000000 ) ) ;
#57213=CARTESIAN_POINT ( 'NONE',  ( 9.269761168585562316, 73.85903009410975528, 118.1934132596428668 ) ) ;
#57217=ORIENTED_EDGE ( 'NONE', *, *, #11600, .F. ) ;
#57237=CARTESIAN_POINT ( 'NONE',  ( -34.75390121890993811, 65.59999999999998010, 71.80362806563780964 ) ) ;
#57249=EDGE_LOOP ( 'NONE', ( #51831, #84591, #85537, #42606, #82597 ) ) ;
#57262=DIRECTION ( 'NONE',  ( 1.821299053822143307E-16, 0.000000000000000000, -1.000000000000000000 ) ) ;
#57304=B_SPLINE_CURVE_WITH_KNOTS ( 'NONE', 3,
 ( #1236, #89833, #29387, #22579, #57068, #71179, #49806, #62992, #70267, #69825, #62551, #50251 ),
 .UNSPECIFIED., .F., .F.,
 ( 4, 2, 2, 2, 2, 4 ),
 ( 0.000000000000000000, 0.0008380503122013481217, 0.001676100624402696243, 0.002514150936604044474, 0.002933176092704727154, 0.003352201248805410268 ),
 .UNSPECIFIED. ) ;
#57319=AXIS2_PLACEMENT_3D ( 'NONE', #8819, #632, #56025 ) ;
#57347=( NAMED_UNIT ( * ) PLANE_ANGLE_UNIT ( ) SI_UNIT ( $, .RADIAN. ) );
#57355=CARTESIAN_POINT ( 'NONE',  ( 0.000000000000000000, 92.07499999999998863, 0.000000000000000000 ) ) ;
#57359=DIRECTION ( 'NONE',  ( -0.9130365726098601531, 0.000000000000000000, -0.4078776986755214828 ) ) ;
#57374=CARTESIAN_POINT ( 'NONE',  ( 0.000000000000000000, 65.60000000000000853, 0.000000000000000000 ) ) ;
#57393=VECTOR ( 'NONE', #34484, 1000.000000000000000 ) ;
#57398=DIRECTION ( 'NONE',  ( -1.000000000000000000, 0.000000000000000000, 0.000000000000000000 ) ) ;
#57412=DIRECTION ( 'NONE',  ( -0.000000000000000000, -1.000000000000000000, -0.000000000000000000 ) ) ;
#57422=ORIENTED_EDGE ( 'NONE', *, *, #71493, .T. ) ;
#57423=ORIENTED_EDGE ( 'NONE', *, *, #22345, .T. ) ;
#57566=CARTESIAN_POINT ( 'NONE',  ( -47.02966122971771767, 65.60000000000000853, -44.00307561052230199 ) ) ;
#57573=LINE ( 'NONE', #71672, #61206 ) ;
#57597=EDGE_LOOP ( 'NONE', ( #41703, #59990, #46248, #88495, #75448 ) ) ;
#57615=DIRECTION ( 'NONE',  ( 0.000000000000000000, 0.000000000000000000, 1.000000000000000000 ) ) ;
#57646=PLANE ( 'NONE',  #81539 ) ;
#57649=CARTESIAN_POINT ( 'NONE',  ( -48.02966122971777452, 65.60000000000000853, 106.4272185163641780 ) ) ;
#57667=VERTEX_POINT ( 'NONE', #51001 ) ;
#57668=AXIS2_PLACEMENT_3D ( 'NONE', #3063, #11667, #24842 ) ;
#57671=AXIS2_PLACEMENT_3D ( 'NONE', #76221, #12661, #33541 ) ;
#57699=PLANE ( 'NONE',  #51918 ) ;
#57732=AXIS2_PLACEMENT_3D ( 'NONE', #69541, #26847, #7317 ) ;
#57746=EDGE_LOOP ( 'NONE', ( #32227, #67692 ) ) ;
#57760=CARTESIAN_POINT ( 'NONE',  ( 12.27784944810749401, 79.68881837611452568, 117.7174742578267370 ) ) ;
#57774=DIRECTION ( 'NONE',  ( -1.000000000000000000, 0.000000000000000000, 0.000000000000000000 ) ) ;
#57777=AXIS2_PLACEMENT_3D ( 'NONE', #81204, #55560, #39829 ) ;
#57781=ORIENTED_EDGE ( 'NONE', *, *, #34638, .F. ) ;
#57791=ORIENTED_EDGE ( 'NONE', *, *, #60031, .T. ) ;
#57795=DIRECTION ( 'NONE',  ( 0.000000000000000000, 0.000000000000000000, 1.000000000000000000 ) ) ;
#57805=LINE ( 'NONE', #10992, #89831 ) ;
#57812=EDGE_CURVE ( 'NONE', #63160, #85945, #68225, .T. ) ;
#57849=FACE_OUTER_BOUND ( 'NONE', #84714, .T. ) ;
#57860=EDGE_LOOP ( 'NONE', ( #44919, #29731, #43022, #6804 ) ) ;
#57871=PLANE ( 'NONE',  #27181 ) ;
#57886=CONICAL_SURFACE ( 'NONE', #69500, 16.33514202138210791, 0.7853981633974552734 ) ;
#57892=VERTEX_POINT ( 'NONE', #53657 ) ;
#57939=EDGE_LOOP ( 'NONE', ( #33863, #52503, #89278, #39980 ) ) ;
#57950=EDGE_LOOP ( 'NONE', ( #4483, #37206 ) ) ;
#57951=VECTOR ( 'NONE', #16530, 999.9999999999998863 ) ;
#58034=AXIS2_PLACEMENT_3D ( 'NONE', #11583, #39274, #4759 ) ;
#58042=ADVANCED_FACE ( 'NONE', ( #34584 ), #62288, .F. ) ;
#58065=CYLINDRICAL_SURFACE ( 'NONE', #31776, 3.814291549405317117 ) ;
#58084=EDGE_CURVE ( 'NONE', #19430, #55378, #86327, .T. ) ;
#58100=EDGE_CURVE ( 'NONE', #77207, #11788, #15948, .T. ) ;
#58138=VERTEX_POINT ( 'NONE', #37734 ) ;
#58157=CARTESIAN_POINT ( 'NONE',  ( -12.17234564962928012, 79.26918314695168988, 117.7284643969750135 ) ) ;
#58172=AXIS2_PLACEMENT_3D ( 'NONE', #31631, #68407, #19806 ) ;
#58204=LINE ( 'NONE', #59521, #12812 ) ;
#58224=CIRCLE ( 'NONE', #65485, 12.60000000000000142 ) ;
#58301=CARTESIAN_POINT ( 'NONE',  ( -544.5124999999999318, 53.97500000000000142, 87.37599999999999056 ) ) ;
#58318=FACE_OUTER_BOUND ( 'NONE', #76800, .T. ) ;
#58319=VERTEX_POINT ( 'NONE', #54442 ) ;
#58349=EDGE_CURVE ( 'NONE', #16953, #34506, #67442, .T. ) ;
#58355=EDGE_CURVE ( 'NONE', #52044, #31278, #25879, .T. ) ;
#58365=DIRECTION ( 'NONE',  ( 0.000000000000000000, 1.000000000000000000, 1.809101308280369915E-15 ) ) ;
#58404=PLANE ( 'NONE',  #11169 ) ;
#58417=DIRECTION ( 'NONE',  ( 0.000000000000000000, 0.000000000000000000, 1.000000000000000000 ) ) ;
#58428=CARTESIAN_POINT ( 'NONE',  ( 69.63919639214307722, 92.07499999999998863, -53.63573739454432854 ) ) ;
#58430=ORIENTED_EDGE ( 'NONE', *, *, #21504, .T. ) ;
#58436=EDGE_LOOP ( 'NONE', ( #50365, #78962, #53109, #83694, #17272, #62479 ) ) ;
#58450=CARTESIAN_POINT ( 'NONE',  ( 70.63919639214310564, 49.07499999999999574, -33.74458626278666884 ) ) ;
#58497=EDGE_LOOP ( 'NONE', ( #54245, #52031, #55270, #70731, #86151 ) ) ;
#58549=CARTESIAN_POINT ( 'NONE',  ( -48.02966122971776741, 93.07500000000001705, 75.53254848357481421 ) ) ;
#58552=LINE ( 'NONE', #65387, #21584 ) ;
#58629=CARTESIAN_POINT ( 'NONE',  ( 12.02669652733116123, 86.65134610876239663, 117.9444722473752307 ) ) ;
#58636=EDGE_CURVE ( 'NONE', #34120, #77564, #25360, .T. ) ;
#58725=DIRECTION ( 'NONE',  ( 1.000000000000000000, 0.000000000000000000, 0.000000000000000000 ) ) ;
#58778=ORIENTED_EDGE ( 'NONE', *, *, #7852, .T. ) ;
#58795=EDGE_CURVE ( 'NONE', #19810, #46234, #74775, .T. ) ;
#58812=FACE_OUTER_BOUND ( 'NONE', #69861, .T. ) ;
#58815=AXIS2_PLACEMENT_3D ( 'NONE', #29251, #56936, #49218 ) ;
#58817=AXIS2_PLACEMENT_3D ( 'NONE', #2269, #84510, #22717 ) ;
#58820=EDGE_CURVE ( 'NONE', #36325, #53045, #25430, .T. ) ;
#58884=ORIENTED_EDGE ( 'NONE', *, *, #69808, .T. ) ;
#58893=LINE ( 'NONE', #39791, #26041 ) ;
#58901=EDGE_LOOP ( 'NONE', ( #69879, #28185, #20690, #5686 ) ) ;
#58933=VECTOR ( 'NONE', #15536, 1000.000000000000000 ) ;
#58967=CARTESIAN_POINT ( 'NONE',  ( -240.5296158183964792, 93.66249999999999432, 90.48749999999999716 ) ) ;
#59012=CARTESIAN_POINT ( 'NONE',  ( -31.27367473141074683, 64.60000000000000853, 74.45358409497265484 ) ) ;
#59027=CARTESIAN_POINT ( 'NONE',  ( -462.0260000000000105, 53.97500000000000142, -3.174999999999999822 ) ) ;
#59039=FACE_OUTER_BOUND ( 'NONE', #78895, .T. ) ;
#59045=ORIENTED_EDGE ( 'NONE', *, *, #9194, .F. ) ;
#59064=ORIENTED_EDGE ( 'NONE', *, *, #62097, .F. ) ;
#59065=DIRECTION ( 'NONE',  ( 0.000000000000000000, -1.000000000000000000, 0.000000000000000000 ) ) ;
#59076=FACE_OUTER_BOUND ( 'NONE', #30914, .T. ) ;
#59106=VERTEX_POINT ( 'NONE', #61841 ) ;
#59124=CARTESIAN_POINT ( 'NONE',  ( -17.13243906362141900, 54.97499999999996589, 42.79834678115690849 ) ) ;
#59176=FACE_BOUND ( 'NONE', #66599, .T. ) ;
#59180=LINE ( 'NONE', #23366, #57951 ) ;
#59204=CARTESIAN_POINT ( 'NONE',  ( -21.42842094847162926, 53.97499999999997300, 41.97446389704172987 ) ) ;
#59211=CIRCLE ( 'NONE', #20076, 11.17600000000001970 ) ;
#59235=CARTESIAN_POINT ( 'NONE',  ( -41.60202597009397607, 65.59999999999998010, 50.85338361873603219 ) ) ;
#59244=DIRECTION ( 'NONE',  ( -0.5000000000000129896, -0.8660254037844311581, 0.000000000000000000 ) ) ;
#59251=DIRECTION ( 'NONE',  ( 0.000000000000000000, 0.000000000000000000, -1.000000000000000000 ) ) ;
#59285=DIRECTION ( 'NONE',  ( 0.000000000000000000, -0.4999999999999928946, -0.8660254037844428154 ) ) ;
#59304=CARTESIAN_POINT ( 'NONE',  ( 68.86456684384336313, 93.07500000000001705, 56.22171674193015889 ) ) ;
#59325=EDGE_CURVE ( 'NONE', #970, #87454, #72265, .T. ) ;
#59381=DIRECTION ( 'NONE',  ( 0.000000000000000000, 1.000000000000000000, 0.000000000000000000 ) ) ;
#59383=ORIENTED_EDGE ( 'NONE', *, *, #43001, .T. ) ;
#59384=VERTEX_POINT ( 'NONE', #79089 ) ;
#59399=VECTOR ( 'NONE', #27496, 1000.000000000000000 ) ;
#59408=CARTESIAN_POINT ( 'NONE',  ( -3.286364562888697272, 94.82452044211723319, 118.5111154470731520 ) ) ;
#59422=DIRECTION ( 'NONE',  ( 0.000000000000000000, -1.000000000000000000, 0.000000000000000000 ) ) ;
#59435=ORIENTED_EDGE ( 'NONE', *, *, #7824, .F. ) ;
#59441=ORIENTED_EDGE ( 'NONE', *, *, #19785, .F. ) ;
#59445=AXIS2_PLACEMENT_3D ( 'NONE', #81618, #19368, #21499 ) ;
#59490=( BOUNDED_CURVE ( )  B_SPLINE_CURVE ( 3, ( #26919, #47792, #55043, #20116 ),
 .UNSPECIFIED., .F., .T. ) 
 B_SPLINE_CURVE_WITH_KNOTS ( ( 4, 4 ),
 ( 1.162083553109172218, 1.162891078689471280 ),
 .UNSPECIFIED. ) 
 CURVE ( )  GEOMETRIC_REPRESENTATION_ITEM ( )  RATIONAL_B_SPLINE_CURVE ( ( 1.000000000000000000, 0.9999999456585371149, 0.9999999456585371149, 1.000000000000000000 ) ) 
 REPRESENTATION_ITEM ( '' )  );
#59499=LINE ( 'NONE', #26776, #40194 ) ;
#59501=EDGE_CURVE ( 'NONE', #24430, #49775, #5453, .T. ) ;
#59502=ORIENTED_EDGE ( 'NONE', *, *, #46250, .T. ) ;
#59518=CARTESIAN_POINT ( 'NONE',  ( 12.19523432446486666, 85.82332710845591350, 117.7261451817823001 ) ) ;
#59521=CARTESIAN_POINT ( 'NONE',  ( -479.3614999999999782, 14.28750000000036025, 2.863608028952925100 ) ) ;
#59531=ORIENTED_EDGE ( 'NONE', *, *, #2141, .F. ) ;
#59539=DIRECTION ( 'NONE',  ( 0.000000000000000000, 1.365923996832131856E-16, -1.000000000000000000 ) ) ;
#59560=VECTOR ( 'NONE', #69905, 1000.000000000000000 ) ;
#59587=EDGE_CURVE ( 'NONE', #58319, #12332, #53961, .T. ) ;
#59594=FACE_OUTER_BOUND ( 'NONE', #55399, .T. ) ;
#59608=ORIENTED_EDGE ( 'NONE', *, *, #14839, .F. ) ;
#59609=VERTEX_POINT ( 'NONE', #7246 ) ;
#59617=EDGE_CURVE ( 'NONE', #22947, #54103, #56254, .T. ) ;
#59649=CARTESIAN_POINT ( 'NONE',  ( -41.60202597009397607, 65.59999999999998010, 47.03909206933071374 ) ) ;
#59659=CARTESIAN_POINT ( 'NONE',  ( -487.2989999999999782, 18.41194598552324990, 83.34375000000000000 ) ) ;
#59680=CARTESIAN_POINT ( 'NONE',  ( -34.53140813619931748, 148.4450814996825443, 35.02576496182814481 ) ) ;
#59752=CARTESIAN_POINT ( 'NONE',  ( -24.20305689751608824, 65.59999999999998010, 58.62596543806478877 ) ) ;
#59774=LINE ( 'NONE', #66146, #82833 ) ;
#59776=CARTESIAN_POINT ( 'NONE',  ( -48.02966122971777452, 100.5999999999999659, 106.4272185163641780 ) ) ;
#59778=ORIENTED_EDGE ( 'NONE', *, *, #61882, .T. ) ;
#59795=ORIENTED_EDGE ( 'NONE', *, *, #17109, .T. ) ;
#59801=ORIENTED_EDGE ( 'NONE', *, *, #40947, .T. ) ;
#59837=CIRCLE ( 'NONE', #64212, 10.00000000000000178 ) ;
#59849=CARTESIAN_POINT ( 'NONE',  ( -4.481496500578191267, 94.44030975666426286, 118.4718929279777200 ) ) ;
#59911=CARTESIAN_POINT ( 'NONE',  ( 69.63919639214310564, 101.5999999999999943, 94.70900412239863897 ) ) ;
#59950=CARTESIAN_POINT ( 'NONE',  ( -34.53140813619931748, 64.60000000000000853, 35.02576496182814481 ) ) ;
#59957=LINE ( 'NONE', #74505, #68749 ) ;
#59960=ORIENTED_EDGE ( 'NONE', *, *, #71445, .F. ) ;
#59966=FACE_OUTER_BOUND ( 'NONE', #13991, .T. ) ;
#59969=CARTESIAN_POINT ( 'NONE',  ( 2.860923566319202305, 70.27222073148661252, 118.3221038006948902 ) ) ;
#59986=ORIENTED_EDGE ( 'NONE', *, *, #280, .T. ) ;
#59990=ORIENTED_EDGE ( 'NONE', *, *, #83008, .F. ) ;
#59991=AXIS2_PLACEMENT_3D ( 'NONE', #36996, #64703, #31496 ) ;
#60031=EDGE_CURVE ( 'NONE', #31377, #17700, #88434, .T. ) ;
#60067=CARTESIAN_POINT ( 'NONE',  ( 70.63919639214310564, 100.5999999999999659, 95.21359708083839735 ) ) ;
#60091=CARTESIAN_POINT ( 'NONE',  ( -446.0240000000000009, 14.28749999999982201, 95.25000000000000000 ) ) ;
#60095=ORIENTED_EDGE ( 'NONE', *, *, #42537, .T. ) ;
#60154=CARTESIAN_POINT ( 'NONE',  ( -479.3614999999999782, 22.53639197104660141, 90.48749999999999716 ) ) ;
#60157=EDGE_CURVE ( 'NONE', #85945, #6718, #85112, .T. ) ;
#60166=ORIENTED_EDGE ( 'NONE', *, *, #85627, .T. ) ;
#60181=ORIENTED_EDGE ( 'NONE', *, *, #7024, .F. ) ;
#60207=ADVANCED_FACE ( 'NONE', ( #83403 ), #21179, .F. ) ;
#60229=EDGE_LOOP ( 'NONE', ( #58778, #15286 ) ) ;
#60235=VECTOR ( 'NONE', #14098, 1000.000000000000114 ) ;
#60260=CARTESIAN_POINT ( 'NONE',  ( -15.88716625750469902, 65.60000000000000853, -53.54073290201169044 ) ) ;
#60266=ORIENTED_EDGE ( 'NONE', *, *, #80033, .T. ) ;
#60282=FACE_OUTER_BOUND ( 'NONE', #51315, .T. ) ;
#60285=LINE ( 'NONE', #13500, #17978 ) ;
#60302=DIRECTION ( 'NONE',  ( 0.000000000000000000, -8.792068030499130893E-15, 1.000000000000000000 ) ) ;
#60324=ADVANCED_FACE ( 'NONE', ( #2077 ), #9334, .F. ) ;
#60338=FACE_OUTER_BOUND ( 'NONE', #54822, .T. ) ;
#60358=CARTESIAN_POINT ( 'NONE',  ( -479.3614999999999782, 18.41194598552324990, 83.34375000000000000 ) ) ;
#60433=ORIENTED_EDGE ( 'NONE', *, *, #75535, .T. ) ;
#60461=ORIENTED_EDGE ( 'NONE', *, *, #68160, .T. ) ;
#60473=CARTESIAN_POINT ( 'NONE',  ( -492.0614999999999668, 93.66249999999999432, 11.11250000000040217 ) ) ;
#60478=ORIENTED_EDGE ( 'NONE', *, *, #17403, .T. ) ;
#60515=CARTESIAN_POINT ( 'NONE',  ( 70.63919639214310564, 91.07499999999996021, -53.97512327982435210 ) ) ;
#60571=AXIS2_PLACEMENT_3D ( 'NONE', #34430, #89873, #27623 ) ;
#60580=CARTESIAN_POINT ( 'NONE',  ( -47.18030668273772221, 100.5999999999999659, 75.34738655934135920 ) ) ;
#60589=LINE ( 'NONE', #88331, #38483 ) ;
#60590=ORIENTED_EDGE ( 'NONE', *, *, #78941, .F. ) ;
#60600=EDGE_CURVE ( 'NONE', #36007, #1586, #50323, .T. ) ;
#60638=FACE_OUTER_BOUND ( 'NONE', #7775, .T. ) ;
#60694=VECTOR ( 'NONE', #67699, 1000.000000000000000 ) ;
#60727=EDGE_LOOP ( 'NONE', ( #41768, #5289, #12677, #83697 ) ) ;
#60753=CARTESIAN_POINT ( 'NONE',  ( -12.03126724623370336, 86.63797872897063712, 117.9440057874066099 ) ) ;
#60827=VERTEX_POINT ( 'NONE', #21976 ) ;
#60883=AXIS2_PLACEMENT_3D ( 'NONE', #78435, #72923, #2568 ) ;
#60889=ORIENTED_EDGE ( 'NONE', *, *, #14144, .T. ) ;
#60900=CARTESIAN_POINT ( 'NONE',  ( -492.0614999999999668, 14.28749999999982201, 90.48749999999999716 ) ) ;
#60908=ORIENTED_EDGE ( 'NONE', *, *, #23034, .F. ) ;
#60931=VERTEX_POINT ( 'NONE', #31888 ) ;
#60939=CARTESIAN_POINT ( 'NONE',  ( -41.60202597009397607, 54.97499999999995879, 50.85338361873603219 ) ) ;
#60957=LINE ( 'NONE', #52757, #54401 ) ;
#60980=LINE ( 'NONE', #11946, #17096 ) ;
#60994=CARTESIAN_POINT ( 'NONE',  ( -10.24823410656255263, 89.89188270629901467, 117.9117007251406335 ) ) ;
#61004=CARTESIAN_POINT ( 'NONE',  ( -24.20305689751608824, 65.59999999999998010, 58.62596543806478877 ) ) ;
#61006=ADVANCED_FACE ( 'NONE', ( #18713 ), #67769, .F. ) ;
#61037=AXIS2_PLACEMENT_3D ( 'NONE', #37788, #16011, #23293 ) ;
#61070=CARTESIAN_POINT ( 'NONE',  ( -47.10523785009519315, 92.57489729980497373, 74.80399995790345713 ) ) ;
#61085=ADVANCED_FACE ( 'NONE', ( #89107 ), #67299, .F. ) ;
#61086=AXIS2_PLACEMENT_3D ( 'NONE', #57096, #22609, #29868 ) ;
#61111=VECTOR ( 'NONE', #55437, 1000.000000000000000 ) ;
#61127=CARTESIAN_POINT ( 'NONE',  ( -479.3614999999999782, 3.174999999999999822, -1.387778780781445991E-14 ) ) ;
#61206=VECTOR ( 'NONE', #22186, 1000.000000000000000 ) ;
#61212=ORIENTED_EDGE ( 'NONE', *, *, #1209, .F. ) ;
#61243=EDGE_CURVE ( 'NONE', #35189, #7001, #64536, .T. ) ;
#61277=DIRECTION ( 'NONE',  ( -0.7071067811865376918, 0.7071067811865574537, -9.811119821538231114E-14 ) ) ;
#61285=ORIENTED_EDGE ( 'NONE', *, *, #19115, .T. ) ;
#61292=VECTOR ( 'NONE', #1312, 1000.000000000000000 ) ;
#61355=EDGE_LOOP ( 'NONE', ( #81658, #88864, #70822, #38598 ) ) ;
#61359=VECTOR ( 'NONE', #8932, 1000.000000000000000 ) ;
#61364=DIRECTION ( 'NONE',  ( -0.7071067811865561215, 0.000000000000000000, 0.7071067811865389130 ) ) ;
#61389=DIRECTION ( 'NONE',  ( 0.000000000000000000, 0.7071067811865401342, 0.7071067811865549002 ) ) ;
#61400=CARTESIAN_POINT ( 'NONE',  ( -24.20305689751608824, 53.97499999999997300, 58.62596543806478877 ) ) ;
#61436=PLANE ( 'NONE',  #26071 ) ;
#61453=ADVANCED_FACE ( 'NONE', ( #85889 ), #16834, .T. ) ;
#61496=CARTESIAN_POINT ( 'NONE',  ( -446.0240000000000009, 14.28750000000026077, 11.11249999999970051 ) ) ;
#61520=AXIS2_PLACEMENT_3D ( 'NONE', #18691, #32766, #3722 ) ;
#61527=ORIENTED_EDGE ( 'NONE', *, *, #43555, .F. ) ;
#61584=FACE_OUTER_BOUND ( 'NONE', #14965, .T. ) ;
#61592=DIRECTION ( 'NONE',  ( -0.7071067811865573427, -0.7071067811865376918, 0.000000000000000000 ) ) ;
#61595=EDGE_LOOP ( 'NONE', ( #9686, #63502, #1268, #26161, #2892, #19218 ) ) ;
#61599=DIRECTION ( 'NONE',  ( 0.000000000000000000, 0.5000000000000012212, -0.8660254037844380415 ) ) ;
#61605=ORIENTED_EDGE ( 'NONE', *, *, #771, .F. ) ;
#61614=ORIENTED_EDGE ( 'NONE', *, *, #43533, .T. ) ;
#61627=EDGE_CURVE ( 'NONE', #72160, #41798, #35361, .T. ) ;
#61652=CARTESIAN_POINT ( 'NONE',  ( -47.05885865011399005, 101.2667695899395426, 108.0895340666595672 ) ) ;
#61660=CIRCLE ( 'NONE', #36983, 118.5560000000000116 ) ;
#61686=CARTESIAN_POINT ( 'NONE',  ( 69.04425121814171007, 92.85005066824639641, 55.64382071430165411 ) ) ;
#61703=VERTEX_POINT ( 'NONE', #10787 ) ;
#61708=EDGE_LOOP ( 'NONE', ( #73840, #80832 ) ) ;
#61730=CARTESIAN_POINT ( 'NONE',  ( -446.0240000000000009, 14.28749999999982201, 90.48749999999999716 ) ) ;
#61740=CIRCLE ( 'NONE', #86416, 4.762500000000002842 ) ;
#61741=DIRECTION ( 'NONE',  ( 0.000000000000000000, 0.000000000000000000, 1.000000000000000000 ) ) ;
#61746=VECTOR ( 'NONE', #8232, 1000.000000000000000 ) ;
#61760=LINE ( 'NONE', #47684, #38945 ) ;
#61762=DIRECTION ( 'NONE',  ( -0.000000000000000000, -1.000000000000000000, 0.000000000000000000 ) ) ;
#61808=CARTESIAN_POINT ( 'NONE',  ( -24.20305689751608824, 53.97499999999997300, 74.96110745944689313 ) ) ;
#61841=CARTESIAN_POINT ( 'NONE',  ( -479.3614999999999782, 3.174999999999999822, -1.387778780781445991E-14 ) ) ;
#61863=CARTESIAN_POINT ( 'NONE',  ( -254.0000000000000000, 3.174999999999999822, 142.8750000000000000 ) ) ;
#61868=ORIENTED_EDGE ( 'NONE', *, *, #4068, .T. ) ;
#61879=CLOSED_SHELL ( 'NONE', ( #5843, #61453, #88680, #16379, #43049, #84905, #21487, #61006, #77071, #43508, #30713, #787, #62103, #66129, #69674, #29804, #1709, #35739, #10925, #46988, #26393, #2006, #65220, #69362, #85052, #80568, #69731, #23664, #72, #61085, #87598, #52427, #47921, #83639, #77693, #33088, #87226, #69791, #63529, #26581, #87233, #13789, #60207, #68872, #1848, #48536, #28667, #88378, #82546, #85689, #85119, #4706, #75129, #46165, #6966, #24658, #7595, #44143, #72131, #60324, #62713, #40353, #55802, #63351, #28349, #56787, #54941, #20777, #36174, #80571, #77915, #22523, #47608, #688, #62301, #82223, #24251, #66382, #48447, #72169, #3853, #20467, #8847, #63017, #27654, #88925, #86911, #86678, #49276, #23492, #7245, #86339, #18704, #88030, #79457, #74922, #64486, #83690, #48378, #52518, #17533, #61913, #35033, #73270, #35524, #72568, #24649, #30482, #6341, #70821, #31302, #23565, #4366, #58042, #52003, #31131, #32187, #21440, #68576, #88846, #44651, #86690, #89688, #75855, #6272, #53347, #74586, #55423, #86433, #20655, #7447, #88565, #88346, #32153, #67421, #73476, #55683, #47206, #52631, #27320, #67986, #22700, #32680, #77690, #27522, #37891, #37715, #26923, #36973, #56604, #10321, #67389, #66569, #86299 ) ) ;
#61882=EDGE_CURVE ( 'NONE', #877, #274, #35996, .T. ) ;
#61908=PLANE ( 'NONE',  #40286 ) ;
#61913=ADVANCED_FACE ( 'NONE', ( #74369 ), #46637, .F. ) ;
#61943=LINE ( 'NONE', #6992, #69310 ) ;
#61945=DIRECTION ( 'NONE',  ( 0.000000000000000000, 0.000000000000000000, -1.000000000000000000 ) ) ;
#61947=FACE_BOUND ( 'NONE', #2027, .T. ) ;
#61954=DIRECTION ( 'NONE',  ( 0.000000000000000000, -0.8660254037844394848, 0.4999999999999986122 ) ) ;
#61980=ORIENTED_EDGE ( 'NONE', *, *, #41349, .F. ) ;
#61999=ORIENTED_EDGE ( 'NONE', *, *, #2024, .F. ) ;
#62043=ORIENTED_EDGE ( 'NONE', *, *, #70130, .F. ) ;
#62080=EDGE_LOOP ( 'NONE', ( #3230, #19933, #64965, #24691 ) ) ;
#62097=EDGE_CURVE ( 'NONE', #78672, #69100, #14721, .T. ) ;
#62103=ADVANCED_FACE ( 'NONE', ( #71917 ), #9681, .T. ) ;
#62117=DIRECTION ( 'NONE',  ( 1.000000000000000000, 0.000000000000000000, 0.000000000000000000 ) ) ;
#62130=FACE_OUTER_BOUND ( 'NONE', #24806, .T. ) ;
#62145=CARTESIAN_POINT ( 'NONE',  ( 68.95544620396594837, 92.96280207012202368, 55.93298909936185481 ) ) ;
#62157=PLANE ( 'NONE',  #73190 ) ;
#62158=ORIENTED_EDGE ( 'NONE', *, *, #27037, .T. ) ;
#62161=CARTESIAN_POINT ( 'NONE',  ( -240.5296158183964792, 14.28750000000026077, 11.11249999999970051 ) ) ;
#62193=CARTESIAN_POINT ( 'NONE',  ( 50.24780502318014896, 92.07499999999998863, -72.12189744004568581 ) ) ;
#62216=ORIENTED_EDGE ( 'NONE', *, *, #9029, .F. ) ;
#62224=CIRCLE ( 'NONE', #11397, 38.10000000000000853 ) ;
#62234=ORIENTED_EDGE ( 'NONE', *, *, #64790, .F. ) ;
#62242=ORIENTED_EDGE ( 'NONE', *, *, #13910, .F. ) ;
#62243=CARTESIAN_POINT ( 'NONE',  ( 1.653928925557865748, 69.93042650361837786, 118.5473008259350678 ) ) ;
#62260=VECTOR ( 'NONE', #1822, 1000.000000000000000 ) ;
#62288=PLANE ( 'NONE',  #29651 ) ;
#62301=ADVANCED_FACE ( 'NONE', ( #45508 ), #31899, .F. ) ;
#62317=EDGE_CURVE ( 'NONE', #47865, #7646, #73230, .T. ) ;
#62359=VECTOR ( 'NONE', #34156, 1000.000000000000000 ) ;
#62379=FACE_OUTER_BOUND ( 'NONE', #66920, .T. ) ;
#62396=DIRECTION ( 'NONE',  ( 0.000000000000000000, 1.000000000000000000, -2.731847993664264698E-16 ) ) ;
#62421=VERTEX_POINT ( 'NONE', #19619 ) ;
#62429=VECTOR ( 'NONE', #5921, 1000.000000000000000 ) ;
#62437=ORIENTED_EDGE ( 'NONE', *, *, #30016, .T. ) ;
#62458=MECHANICAL_DESIGN_GEOMETRIC_PRESENTATION_REPRESENTATION('',(#24725),#30374);
#62479=ORIENTED_EDGE ( 'NONE', *, *, #14144, .F. ) ;
#62496=CARTESIAN_POINT ( 'NONE',  ( -40.89999999999999858, 53.97500000000000142, 40.79999999999999716 ) ) ;
#62514=DIRECTION ( 'NONE',  ( 0.9130365726098601531, 0.000000000000000000, 0.4078776986755214828 ) ) ;
#62522=EDGE_LOOP ( 'NONE', ( #76603, #21278, #82829, #5623, #88877, #77900 ) ) ;
#62533=EDGE_CURVE ( 'NONE', #8809, #15378, #84107, .T. ) ;
#62551=CARTESIAN_POINT ( 'NONE',  ( -55.94501007020270578, 55.83380253633427515, 70.71393962117267051 ) ) ;
#62594=CARTESIAN_POINT ( 'NONE',  ( 69.21917243687391874, 92.62461542576163254, 55.06468400917383832 ) ) ;
#62596=EDGE_CURVE ( 'NONE', #16017, #82548, #12862, .T. ) ;
#62612=PRODUCT_DEFINITION_CONTEXT ( 'detailed design', #18985, 'design' ) ;
#62618=CARTESIAN_POINT ( 'NONE',  ( -546.0365000000000464, 53.97500000000000142, 87.37599999999999056 ) ) ;
#62641=FACE_OUTER_BOUND ( 'NONE', #29626, .T. ) ;
#62673=CIRCLE ( 'NONE', #85914, 4.762500000000002842 ) ;
#62689=DIRECTION ( 'NONE',  ( 0.000000000000000000, 0.000000000000000000, 1.000000000000000000 ) ) ;
#62699=ORIENTED_EDGE ( 'NONE', *, *, #51314, .F. ) ;
#62713=ADVANCED_FACE ( 'NONE', ( #44522 ), #79530, .F. ) ;
#62740=LINE ( 'NONE', #83205, #46565 ) ;
#62774=CARTESIAN_POINT ( 'NONE',  ( -479.3614999999999782, 85.41360802895360393, 11.11250000000036131 ) ) ;
#62779=CARTESIAN_POINT ( 'NONE',  ( -4.055571906748874689, 94.48660284847177593, 118.2871548781509432 ) ) ;
#62785=DIRECTION ( 'NONE',  ( -0.000000000000000000, -1.000000000000000000, -0.000000000000000000 ) ) ;
#62835=ORIENTED_EDGE ( 'NONE', *, *, #73281, .T. ) ;
#62906=CARTESIAN_POINT ( 'NONE',  ( 70.63919639214310564, 65.60000000000000853, 56.85413200336923012 ) ) ;
#62923=EDGE_LOOP ( 'NONE', ( #68993, #31960, #86298, #6071 ) ) ;
#62930=DIRECTION ( 'NONE',  ( -0.000000000000000000, -1.000000000000000000, -0.000000000000000000 ) ) ;
#62984=DIRECTION ( 'NONE',  ( 0.000000000000000000, 1.000000000000000000, 0.000000000000000000 ) ) ;
#62992=CARTESIAN_POINT ( 'NONE',  ( -55.79405894393751453, 55.29575870445238195, 70.75673509094546887 ) ) ;
#63009=EDGE_CURVE ( 'NONE', #72100, #14882, #9041, .T. ) ;
#63017=ADVANCED_FACE ( 'NONE', ( #62641 ), #69915, .T. ) ;
#63019=ORIENTED_EDGE ( 'NONE', *, *, #88559, .F. ) ;
#63052=DIRECTION ( 'NONE',  ( 0.000000000000000000, -1.000000000000000000, -3.491483361109380094E-15 ) ) ;
#63075=CARTESIAN_POINT ( 'NONE',  ( -48.02966122971774610, 66.60000000000003695, -43.00307561052233751 ) ) ;
#63091=PLANE ( 'NONE',  #34169 ) ;
#63115=ADVANCED_FACE ( 'NONE', ( #64890 ), #58065, .F. ) ;
#63122=VECTOR ( 'NONE', #31903, 1000.000000000000000 ) ;
#63134=VERTEX_POINT ( 'NONE', #38070 ) ;
#63137=CARTESIAN_POINT ( 'NONE',  ( -446.0240000000000009, 3.174999999999999822, -1.387778780781445991E-14 ) ) ;
#63146=CARTESIAN_POINT ( 'NONE',  ( 3.292116081692606944, 70.27706896417943483, 118.5109511094031944 ) ) ;
#63160=VERTEX_POINT ( 'NONE', #30808 ) ;
#63223=EDGE_CURVE ( 'NONE', #8859, #59384, #23125, .T. ) ;
#63226=CARTESIAN_POINT ( 'NONE',  ( 6.310004044849506499, 93.46397155878921126, 118.1882387953691591 ) ) ;
#63233=CARTESIAN_POINT ( 'NONE',  ( -487.2989999999999782, 97.78694598552380057, 3.968750000000479616 ) ) ;
#63241=VECTOR ( 'NONE', #56386, 999.9999999999998863 ) ;
#63261=VECTOR ( 'NONE', #49777, 1000.000000000000000 ) ;
#63267=ORIENTED_EDGE ( 'NONE', *, *, #26575, .T. ) ;
#63285=DIRECTION ( 'NONE',  ( -1.000000000000000000, 0.000000000000000000, 0.000000000000000000 ) ) ;
#63286=CARTESIAN_POINT ( 'NONE',  ( -40.89999999999999858, 53.97500000000000142, 60.79999999999999716 ) ) ;
#63301=FACE_OUTER_BOUND ( 'NONE', #45384, .T. ) ;
#63346=DIRECTION ( 'NONE',  ( 0.000000000000000000, 0.000000000000000000, -1.000000000000000000 ) ) ;
#63351=ADVANCED_FACE ( 'NONE', ( #69364 ), #1223, .F. ) ;
#63352=DIRECTION ( 'NONE',  ( -1.000000000000000000, 0.000000000000000000, 0.000000000000000000 ) ) ;
#63359=AXIS2_PLACEMENT_3D ( 'NONE', #48914, #42552, #8058 ) ;
#63382=LINE ( 'NONE', #1164, #37324 ) ;
#63397=LINE ( 'NONE', #83855, #7602 ) ;
#63416=CARTESIAN_POINT ( 'NONE',  ( -41.60202597009397607, 40.59999999999997300, 50.85338361873603219 ) ) ;
#63437=CARTESIAN_POINT ( 'NONE',  ( -50.35902679310718355, 54.97499999999996589, 27.95514712793348977 ) ) ;
#63445=CARTESIAN_POINT ( 'NONE',  ( -6.715534948705635721, 71.76285132298018254, 118.3661493156453730 ) ) ;
#63447=CIRCLE ( 'NONE', #57668, 38.10000000000000142 ) ;
#63493=DIRECTION ( 'NONE',  ( 0.9130365726098600421, 0.000000000000000000, 0.4078776986755216494 ) ) ;
#63499=PLANE ( 'NONE',  #48269 ) ;
#63502=ORIENTED_EDGE ( 'NONE', *, *, #62317, .T. ) ;
#63514=CARTESIAN_POINT ( 'NONE',  ( -254.0000000000000000, 93.66249999999999432, 11.11250000000040217 ) ) ;
#63521=ORIENTED_EDGE ( 'NONE', *, *, #33359, .T. ) ;
#63529=ADVANCED_FACE ( 'NONE', ( #37528 ), #49268, .F. ) ;
#63530=CARTESIAN_POINT ( 'NONE',  ( -458.3598257906459708, 60.32499999999999574, 3.174999999999999822 ) ) ;
#63532=CARTESIAN_POINT ( 'NONE',  ( -41.60202597009397607, 65.59999999999998010, 34.51824159735389941 ) ) ;
#63546=CARTESIAN_POINT ( 'NONE',  ( -75.11741860696075435, 54.02010448448870505, 30.79984509629914768 ) ) ;
#63554=VECTOR ( 'NONE', #74143, 1000.000000000000000 ) ;
#63574=LINE ( 'NONE', #29058, #9534 ) ;
#63601=DIRECTION ( 'NONE',  ( -0.000000000000000000, 1.000000000000000000, -0.000000000000000000 ) ) ;
#63604=ORIENTED_EDGE ( 'NONE', *, *, #44343, .F. ) ;
#63625=ORIENTED_EDGE ( 'NONE', *, *, #35071, .T. ) ;
#63640=CARTESIAN_POINT ( 'NONE',  ( -446.0240000000000009, 53.97500000000000142, 0.000000000000000000 ) ) ;
#63650=EDGE_CURVE ( 'NONE', #72907, #27384, #29210, .T. ) ;
#63673=DIRECTION ( 'NONE',  ( -0.000000000000000000, -1.000000000000000000, 0.000000000000000000 ) ) ;
#63677=CARTESIAN_POINT ( 'NONE',  ( 5.203398961192315042, 94.03281790535285722, 118.2421799489154211 ) ) ;
#63688=AXIS2_PLACEMENT_3D ( 'NONE', #63437, #43422, #48429 ) ;
#63690=AXIS2_PLACEMENT_3D ( 'NONE', #59752, #87486, #36320 ) ;
#63705=AXIS2_PLACEMENT_3D ( 'NONE', #51429, #79177, #2415 ) ;
#63802=AXIS2_PLACEMENT_3D ( 'NONE', #85143, #65997, #71064 ) ;
#63807=ORIENTED_EDGE ( 'NONE', *, *, #61243, .F. ) ;
#63809=VECTOR ( 'NONE', #39629, 1000.000000000000000 ) ;
#63825=DIRECTION ( 'NONE',  ( 0.000000000000000000, 0.000000000000000000, 1.000000000000000000 ) ) ;
#63847=DIRECTION ( 'NONE',  ( 0.000000000000000000, 0.8660254037844428154, -0.4999999999999928946 ) ) ;
#63849=CARTESIAN_POINT ( 'NONE',  ( -47.02966122971771767, 65.60000000000000853, -44.00307561052230199 ) ) ;
#63879=ORIENTED_EDGE ( 'NONE', *, *, #66474, .T. ) ;
#63902=CIRCLE ( 'NONE', #30560, 4.762500000000002842 ) ;
#63914=DIRECTION ( 'NONE',  ( 0.000000000000000000, 0.000000000000000000, -1.000000000000000000 ) ) ;
#63936=CARTESIAN_POINT ( 'NONE',  ( -487.2989999999999782, 97.78694598552370110, 18.25625000000050235 ) ) ;
#63943=EDGE_LOOP ( 'NONE', ( #31866, #28506, #23451, #33874 ) ) ;
#63988=DIRECTION ( 'NONE',  ( -1.000000000000000000, -0.000000000000000000, -0.000000000000000000 ) ) ;
#64002=DIRECTION ( 'NONE',  ( -0.3600166455925385423, -9.815533969194669696E-15, -0.9329458799396118662 ) ) ;
#64036=ORIENTED_EDGE ( 'NONE', *, *, #24278, .F. ) ;
#64046=CARTESIAN_POINT ( 'NONE',  ( 0.000000000000000000, 65.60000000000000853, 0.000000000000000000 ) ) ;
#64050=EDGE_CURVE ( 'NONE', #13441, #76709, #73884, .T. ) ;
#64053=CARTESIAN_POINT ( 'NONE',  ( 12.03224243969232354, 78.46476182159877055, 117.9439065551169108 ) ) ;
#64088=DIRECTION ( 'NONE',  ( 0.000000000000000000, 0.000000000000000000, -1.000000000000000000 ) ) ;
#64095=CIRCLE ( 'NONE', #81478, 4.762500000000002842 ) ;
#64149=EDGE_CURVE ( 'NONE', #30549, #8470, #87523, .T. ) ;
#64160=DIRECTION ( 'NONE',  ( -0.000000000000000000, -1.000000000000000000, -0.000000000000000000 ) ) ;
#64192=LINE ( 'NONE', #2412, #25216 ) ;
#64204=EDGE_CURVE ( 'NONE', #43607, #10009, #20716, .T. ) ;
#64207=CARTESIAN_POINT ( 'NONE',  ( -465.6921742093539933, 60.32499999999999574, 3.174999999999999822 ) ) ;
#64210=DIRECTION ( 'NONE',  ( -0.000000000000000000, 1.000000000000000000, -0.000000000000000000 ) ) ;
#64212=AXIS2_PLACEMENT_3D ( 'NONE', #63286, #27412, #1062 ) ;
#64270=EDGE_CURVE ( 'NONE', #3353, #47865, #47944, .T. ) ;
#64277=VECTOR ( 'NONE', #76541, 1000.000000000000114 ) ;
#64300=CARTESIAN_POINT ( 'NONE',  ( -41.60202597009397607, 53.97499999999997300, 50.85338361873603219 ) ) ;
#64330=CARTESIAN_POINT ( 'NONE',  ( -454.6936515812919879, 53.97500000000000142, 3.174999999999999822 ) ) ;
#64392=FACE_OUTER_BOUND ( 'NONE', #75314, .T. ) ;
#64422=CIRCLE ( 'NONE', #76011, 10.00000000000000178 ) ;
#64438=EDGE_CURVE ( 'NONE', #51309, #8809, #49300, .T. ) ;
#64470=EDGE_CURVE ( 'NONE', #9022, #83591, #86533, .T. ) ;
#64471=B_SPLINE_CURVE_WITH_KNOTS ( 'NONE', 3,
 ( #65119, #42977, #72827, #70717, #10593, #42533, #4232, #86912, #51905, #80107, #63445, #38297, #10158, #25116, #38742, #44659, #86474, #65996, #77530, #9712, #3788, #28934, #37416, #56620, #31475, #2903 ),
 .UNSPECIFIED., .F., .F.,
 ( 4, 2, 2, 2, 2, 2, 2, 2, 2, 2, 2, 2, 4 ),
 ( 0.01987185114512061979, 0.02111326483159428266, 0.02235467851806794207, 0.02483750589101525741, 0.02607891957748890294, 0.02732033326396255193, 0.02980316063690985340, 0.03228598800985715833, 0.03352740169633080386, 0.03476881538280444939, 0.03725164275575171269, 0.03849305644222534434, 0.03973447012869897599 ),
 .UNSPECIFIED. ) ;
#64485=ORIENTED_EDGE ( 'NONE', *, *, #68038, .T. ) ;
#64486=ADVANCED_FACE ( 'NONE', ( #31094 ), #72006, .F. ) ;
#64536=LINE ( 'NONE', #8230, #70703 ) ;
#64542=VECTOR ( 'NONE', #23710, 1000.000000000000114 ) ;
#64560=VERTEX_POINT ( 'NONE', #37030 ) ;
#64575=EDGE_CURVE ( 'NONE', #32749, #49587, #23856, .T. ) ;
#64583=CARTESIAN_POINT ( 'NONE',  ( 8.621919111718908013, 73.35264728006647772, 118.0418996292485190 ) ) ;
#64656=EDGE_CURVE ( 'NONE', #42067, #81257, #1518, .T. ) ;
#64657=EDGE_CURVE ( 'NONE', #45431, #10945, #77361, .T. ) ;
#64663=EDGE_CURVE ( 'NONE', #55378, #50747, #49184, .T. ) ;
#64671=CIRCLE ( 'NONE', #76272, 1.523999999999997579 ) ;
#64682=EDGE_CURVE ( 'NONE', #36722, #19524, #49635, .T. ) ;
#64700=ORIENTED_EDGE ( 'NONE', *, *, #58100, .F. ) ;
#64703=DIRECTION ( 'NONE',  ( -1.000000000000000000, 0.000000000000000000, 0.000000000000000000 ) ) ;
#64708=EDGE_CURVE ( 'NONE', #77564, #34120, #1311, .T. ) ;
#64783=DIRECTION ( 'NONE',  ( -1.776356839400250465E-15, 0.000000000000000000, -1.000000000000000000 ) ) ;
#64790=EDGE_CURVE ( 'NONE', #26777, #33481, #57805, .T. ) ;
#64798=AXIS2_PLACEMENT_3D ( 'NONE', #47850, #5651, #68768 ) ;
#64800=AXIS2_PLACEMENT_3D ( 'NONE', #3020, #17103, #63914 ) ;
#64816=VERTEX_POINT ( 'NONE', #73212 ) ;
#64827=DIRECTION ( 'NONE',  ( -1.000000000000000000, 0.000000000000000000, 0.000000000000000000 ) ) ;
#64831=ORIENTED_EDGE ( 'NONE', *, *, #36681, .F. ) ;
#64832=DIRECTION ( 'NONE',  ( -1.000000000000000000, 0.000000000000000000, 0.000000000000000000 ) ) ;
#64890=FACE_OUTER_BOUND ( 'NONE', #87256, .T. ) ;
#64919=FACE_OUTER_BOUND ( 'NONE', #74449, .T. ) ;
#64940=CIRCLE ( 'NONE', #88231, 10.00000000000000178 ) ;
#64965=ORIENTED_EDGE ( 'NONE', *, *, #1604, .F. ) ;
#64981=CARTESIAN_POINT ( 'NONE',  ( -215.9000000000000057, 104.7749999999999915, -41.27499999999999858 ) ) ;
#65064=LINE ( 'NONE', #70542, #39165 ) ;
#65096=CARTESIAN_POINT ( 'NONE',  ( 68.86456684384336313, 100.5999999999999659, 56.22171674193015889 ) ) ;
#65108=VERTEX_POINT ( 'NONE', #4633 ) ;
#65114=CARTESIAN_POINT ( 'NONE',  ( -446.0240000000000009, 14.28750000000026077, 11.11249999999970051 ) ) ;
#65119=CARTESIAN_POINT ( 'NONE',  ( 1.796236281188243881E-22, 69.84999999999999432, 118.5560000000000116 ) ) ;
#65124=ORIENTED_EDGE ( 'NONE', *, *, #79652, .T. ) ;
#65173=ORIENTED_EDGE ( 'NONE', *, *, #83539, .T. ) ;
#65191=FACE_OUTER_BOUND ( 'NONE', #80077, .T. ) ;
#65198=CYLINDRICAL_SURFACE ( 'NONE', #41616, 4.762500000000000178 ) ;
#65220=ADVANCED_FACE ( 'NONE', ( #27310 ), #75915, .F. ) ;
#65254=FACE_OUTER_BOUND ( 'NONE', #19540, .T. ) ;
#65272=FACE_OUTER_BOUND ( 'NONE', #36299, .T. ) ;
#65280=AXIS2_PLACEMENT_3D ( 'NONE', #28128, #40866, #7702 ) ;
#65365=ORIENTED_EDGE ( 'NONE', *, *, #15525, .F. ) ;
#65370=ORIENTED_EDGE ( 'NONE', *, *, #85922, .T. ) ;
#65377=CARTESIAN_POINT ( 'NONE',  ( -479.3614999999999782, 6.038608028953049711, 90.48749999999999716 ) ) ;
#65387=CARTESIAN_POINT ( 'NONE',  ( -479.3614999999999782, 3.174999999999999822, 101.5999999999999943 ) ) ;
#65423=CARTESIAN_POINT ( 'NONE',  ( -12.59999999999999964, 81.71744534370293422, 117.6834004267381601 ) ) ;
#65445=ORIENTED_EDGE ( 'NONE', *, *, #27127, .F. ) ;
#65446=EDGE_CURVE ( 'NONE', #85611, #43607, #19838, .T. ) ;
#65456=DIRECTION ( 'NONE',  ( -1.000000000000000000, 0.000000000000000000, 0.000000000000000000 ) ) ;
#65463=DIRECTION ( 'NONE',  ( 1.000000000000000000, 0.000000000000000000, 0.000000000000000000 ) ) ;
#65466=CARTESIAN_POINT ( 'NONE',  ( -64.50026246089650783, 54.97499999999996589, 59.61038444174924678 ) ) ;
#65485=AXIS2_PLACEMENT_3D ( 'NONE', #33831, #42417, #207 ) ;
#65558=CARTESIAN_POINT ( 'NONE',  ( -47.02966122971774610, 92.07499999999998863, 74.26049396966043048 ) ) ;
#65563=VECTOR ( 'NONE', #12225, 1000.000000000000000 ) ;
#65570=AXIS2_PLACEMENT_3D ( 'NONE', #30995, #38256, #52295 ) ;
#65584=ORIENTED_EDGE ( 'NONE', *, *, #74407, .T. ) ;
#65586=LINE ( 'NONE', #9293, #68100 ) ;
#65596=ORIENTED_EDGE ( 'NONE', *, *, #73281, .F. ) ;
#65641=DIRECTION ( 'NONE',  ( 0.000000000000000000, -0.000000000000000000, -1.000000000000000000 ) ) ;
#65659=CARTESIAN_POINT ( 'NONE',  ( -487.2989999999999782, 14.28750000000023945, 19.36139197104649767 ) ) ;
#65665=DIRECTION ( 'NONE',  ( 0.000000000000000000, 0.000000000000000000, 1.000000000000000000 ) ) ;
#65715=PLANE ( 'NONE',  #18876 ) ;
#65718=DIRECTION ( 'NONE',  ( 1.000000000000000000, 0.000000000000000000, 0.000000000000000000 ) ) ;
#65744=VERTEX_POINT ( 'NONE', #84771 ) ;
#65750=CARTESIAN_POINT ( 'NONE',  ( -15.89999999999999680, 53.97500000000000142, 50.79999999999999716 ) ) ;
#65774=EDGE_CURVE ( 'NONE', #88630, #49587, #73981, .T. ) ;
#65784=VERTEX_POINT ( 'NONE', #52855 ) ;
#65851=FACE_OUTER_BOUND ( 'NONE', #71529, .T. ) ;
#65865=CARTESIAN_POINT ( 'NONE',  ( -64.50026246089650783, 54.97499999999996589, 59.61038444174924678 ) ) ;
#65917=FACE_OUTER_BOUND ( 'NONE', #48258, .T. ) ;
#65926=EDGE_LOOP ( 'NONE', ( #51102, #77684, #25833, #34372 ) ) ;
#65954=FACE_OUTER_BOUND ( 'NONE', #49578, .T. ) ;
#65956=CARTESIAN_POINT ( 'NONE',  ( -41.60202597009397607, 65.59999999999998010, 33.51824159735392783 ) ) ;
#65986=CIRCLE ( 'NONE', #10887, 3.814291549405317117 ) ;
#65988=EDGE_CURVE ( 'NONE', #13052, #80177, #24635, .T. ) ;
#65996=CARTESIAN_POINT ( 'NONE',  ( -11.39405732433012375, 76.92513621822203618, 118.0073709438022576 ) ) ;
#65997=DIRECTION ( 'NONE',  ( -0.000000000000000000, 1.000000000000000000, -0.000000000000000000 ) ) ;
#66014=ORIENTED_EDGE ( 'NONE', *, *, #36211, .T. ) ;
#66021=AXIS2_PLACEMENT_3D ( 'NONE', #71107, #55183, #76105 ) ;
#66100=PLANE ( 'NONE',  #9424 ) ;
#66114=CARTESIAN_POINT ( 'NONE',  ( -479.3614999999999782, 104.7749999999999915, 101.5999999999999943 ) ) ;
#66120=ORIENTED_EDGE ( 'NONE', *, *, #76853, .F. ) ;
#66129=ADVANCED_FACE ( 'NONE', ( #50099 ), #22425, .F. ) ;
#66134=VECTOR ( 'NONE', #84579, 1000.000000000000000 ) ;
#66135=VECTOR ( 'NONE', #26676, 1000.000000000000000 ) ;
#66144=DIRECTION ( 'NONE',  ( 0.000000000000000000, 0.000000000000000000, 1.000000000000000000 ) ) ;
#66146=CARTESIAN_POINT ( 'NONE',  ( -479.3614999999999782, 21.43125000000035030, 6.988054014476359654 ) ) ;
#66154=PLANE ( 'NONE',  #83820 ) ;
#66155=EDGE_CURVE ( 'NONE', #84840, #39332, #56007, .T. ) ;
#66169=DIRECTION ( 'NONE',  ( -0.7071067811865660024, 8.659560562355160888E-17, 0.7071067811865291430 ) ) ;
#66185=ORIENTED_EDGE ( 'NONE', *, *, #68772, .T. ) ;
#66203=CIRCLE ( 'NONE', #37182, 4.762500000000002842 ) ;
#66221=CARTESIAN_POINT ( 'NONE',  ( -9.568504969587623421, 90.94163949856141471, 118.1706967199356626 ) ) ;
#66222=EDGE_LOOP ( 'NONE', ( #38303, #34290, #66519, #74629, #80265 ) ) ;
#66232=LINE ( 'NONE', #32166, #28505 ) ;
#66236=DIRECTION ( 'NONE',  ( 0.000000000000000000, 1.000000000000000000, 0.000000000000000000 ) ) ;
#66255=ORIENTED_EDGE ( 'NONE', *, *, #77082, .F. ) ;
#66257=CARTESIAN_POINT ( 'NONE',  ( -479.3614999999999782, 100.8062500000000057, 86.36305401447658880 ) ) ;
#66285=FACE_OUTER_BOUND ( 'NONE', #30311, .T. ) ;
#66299=EDGE_LOOP ( 'NONE', ( #16128, #76830, #49033, #53473 ) ) ;
#66301=LINE ( 'NONE', #10897, #480 ) ;
#66323=AXIS2_PLACEMENT_3D ( 'NONE', #39891, #13105, #356 ) ;
#66336=DIRECTION ( 'NONE',  ( 0.000000000000000000, 0.8660254037844379305, 0.5000000000000011102 ) ) ;
#66347=VECTOR ( 'NONE', #37581, 1000.000000000000000 ) ;
#66362=DIRECTION ( 'NONE',  ( -1.000000000000000000, 0.000000000000000000, 0.000000000000000000 ) ) ;
#66382=ADVANCED_FACE ( 'NONE', ( #3313 ), #51436, .T. ) ;
#66427=CARTESIAN_POINT ( 'NONE',  ( -487.2989999999999782, 14.28749999999982201, 95.25000000000000000 ) ) ;
#66436=CIRCLE ( 'NONE', #12773, 4.762500000000000178 ) ;
#66448=ORIENTED_EDGE ( 'NONE', *, *, #28911, .T. ) ;
#66470=VERTEX_POINT ( 'NONE', #19613 ) ;
#66473=CARTESIAN_POINT ( 'NONE',  ( -47.11752803141010304, 65.68786680169236547, 108.7909173056707317 ) ) ;
#66474=EDGE_CURVE ( 'NONE', #86124, #7001, #11464, .T. ) ;
#66482=EDGE_CURVE ( 'NONE', #16780, #10687, #6434, .T. ) ;
#66505=CARTESIAN_POINT ( 'NONE',  ( -240.5296158183964792, 93.66249999999999432, 11.11250000000040217 ) ) ;
#66519=ORIENTED_EDGE ( 'NONE', *, *, #2165, .F. ) ;
#66532=AXIS2_PLACEMENT_3D ( 'NONE', #9141, #36837, #14613 ) ;
#66535=ORIENTED_EDGE ( 'NONE', *, *, #38690, .F. ) ;
#66537=VECTOR ( 'NONE', #34958, 1000.000000000000000 ) ;
#66551=CARTESIAN_POINT ( 'NONE',  ( -240.5296158183964792, 14.28749999999982201, 90.48749999999999716 ) ) ;
#66554=CARTESIAN_POINT ( 'NONE',  ( -487.2989999999999782, 14.28750000000036025, 2.863608028952925100 ) ) ;
#66569=ADVANCED_FACE ( 'NONE', ( #8235 ), #35028, .T. ) ;
#66585=ORIENTED_EDGE ( 'NONE', *, *, #51008, .F. ) ;
#66593=CARTESIAN_POINT ( 'NONE',  ( -446.0240000000000009, 14.28750000000026077, 6.349999999999710099 ) ) ;
#66599=EDGE_LOOP ( 'NONE', ( #10895, #913 ) ) ;
#66608=DIRECTION ( 'NONE',  ( 1.000000000000000000, 0.000000000000000000, 0.000000000000000000 ) ) ;
#66611=FACE_OUTER_BOUND ( 'NONE', #49438, .T. ) ;
#66631=CARTESIAN_POINT ( 'NONE',  ( -487.2989999999999782, 22.53639197104660141, 90.48749999999999716 ) ) ;
#66672=ORIENTED_EDGE ( 'NONE', *, *, #33901, .F. ) ;
#66680=CARTESIAN_POINT ( 'NONE',  ( -12.61954384753730096, 84.20405175638288142, 117.8825647057245192 ) ) ;
#66716=CARTESIAN_POINT ( 'NONE',  ( -48.02966122971776741, 93.07500000000001705, 75.53254848357481421 ) ) ;
#66744=CONICAL_SURFACE ( 'NONE', #7299, 10.41399999999997839, 0.7853981633974744803 ) ;
#66747=ORIENTED_EDGE ( 'NONE', *, *, #19785, .T. ) ;
#66774=VECTOR ( 'NONE', #68668, 1000.000000000000000 ) ;
#66800=DIRECTION ( 'NONE',  ( 0.000000000000000000, -0.8660254037844336006, -0.5000000000000088818 ) ) ;
#66802=LINE ( 'NONE', #24144, #64542 ) ;
#66803=ORIENTED_EDGE ( 'NONE', *, *, #41452, .T. ) ;
#66810=AXIS2_PLACEMENT_3D ( 'NONE', #40437, #61762, #33631 ) ;
#66828=CARTESIAN_POINT ( 'NONE',  ( -215.9000000000000057, 53.97500000000000142, 50.79999999999999716 ) ) ;
#66870=CARTESIAN_POINT ( 'NONE',  ( -469.3583484187089994, 53.97500000000000142, 3.174999999999999822 ) ) ;
#66920=EDGE_LOOP ( 'NONE', ( #56662, #65173, #908, #42667, #23486, #6622 ) ) ;
#66934=EDGE_LOOP ( 'NONE', ( #59441, #84041, #60181, #2230, #68812, #48413, #23988 ) ) ;
#66935=EDGE_LOOP ( 'NONE', ( #63625, #57423, #70674, #57140 ) ) ;
#66960=CYLINDRICAL_SURFACE ( 'NONE', #42044, 4.762500000000001066 ) ;
#66985=ORIENTED_EDGE ( 'NONE', *, *, #43555, .T. ) ;
#67013=ORIENTED_EDGE ( 'NONE', *, *, #73110, .F. ) ;
#67042=VERTEX_POINT ( 'NONE', #63075 ) ;
#67058=DIRECTION ( 'NONE',  ( 0.000000000000000000, -1.000000000000000000, 0.000000000000000000 ) ) ;
#67059=EDGE_CURVE ( 'NONE', #34506, #29469, #6772, .T. ) ;
#67079=FACE_BOUND ( 'NONE', #382, .T. ) ;
#67114=EDGE_CURVE ( 'NONE', #65744, #50718, #48978, .T. ) ;
#67119=DIRECTION ( 'NONE',  ( -1.000000000000000000, 0.000000000000000000, 0.000000000000000000 ) ) ;
#67123=CARTESIAN_POINT ( 'NONE',  ( 0.000000000000000000, 82.54999999999999716, 92.46299999999996544 ) ) ;
#67128=CARTESIAN_POINT ( 'NONE',  ( -0.8397198549841756732, 95.25000000000002842, 118.5560000000000258 ) ) ;
#67146=ORIENTED_EDGE ( 'NONE', *, *, #67555, .T. ) ;
#67171=CIRCLE ( 'NONE', #19133, 12.60000000000000142 ) ;
#67226=AXIS2_PLACEMENT_3D ( 'NONE', #62496, #76586, #56108 ) ;
#67232=DIRECTION ( 'NONE',  ( 0.000000000000000000, -1.000000000000000000, 0.000000000000000000 ) ) ;
#67256=AXIS2_PLACEMENT_3D ( 'NONE', #37080, #2569, #24343 ) ;
#67270=DIRECTION ( 'NONE',  ( -0.000000000000000000, 1.000000000000000000, -0.000000000000000000 ) ) ;
#67295=FACE_OUTER_BOUND ( 'NONE', #28629, .T. ) ;
#67297=DIRECTION ( 'NONE',  ( 1.000000000000000000, 0.000000000000000000, 0.000000000000000000 ) ) ;
#67299=PLANE ( 'NONE',  #69266 ) ;
#67311=DIRECTION ( 'NONE',  ( 0.000000000000000000, -1.000000000000000000, 2.048885995248194949E-16 ) ) ;
#67327=VERTEX_POINT ( 'NONE', #3100 ) ;
#67332=DIRECTION ( 'NONE',  ( -1.000000000000000000, 0.000000000000000000, 0.000000000000000000 ) ) ;
#67354=ORIENTED_EDGE ( 'NONE', *, *, #4194, .T. ) ;
#67389=ADVANCED_FACE ( 'NONE', ( #36278 ), #38062, .T. ) ;
#67415=CARTESIAN_POINT ( 'NONE',  ( -487.2989999999999782, 97.78694598552380057, 3.968750000000479616 ) ) ;
#67418=DIRECTION ( 'NONE',  ( 0.000000000000000000, -1.000000000000000000, 0.000000000000000000 ) ) ;
#67421=ADVANCED_FACE ( 'NONE', ( #18055 ), #88003, .T. ) ;
#67438=ORIENTED_EDGE ( 'NONE', *, *, #33681, .T. ) ;
#67442=CIRCLE ( 'NONE', #83419, 4.762500000000000178 ) ;
#67462=DIRECTION ( 'NONE',  ( 0.000000000000000000, 0.000000000000000000, 1.000000000000000000 ) ) ;
#67465=VECTOR ( 'NONE', #61954, 999.9999999999998863 ) ;
#67495=ORIENTED_EDGE ( 'NONE', *, *, #30932, .F. ) ;
#67530=CARTESIAN_POINT ( 'NONE',  ( 68.86456684384336313, 93.07500000000001705, 56.22171674193015889 ) ) ;
#67543=EDGE_LOOP ( 'NONE', ( #59960, #74420, #59986, #28376, #78660 ) ) ;
#67555=EDGE_CURVE ( 'NONE', #36722, #12182, #26216, .T. ) ;
#67592=CARTESIAN_POINT ( 'NONE',  ( -24.20305689751608824, 54.97499999999995879, 58.62596543806478877 ) ) ;
#67617=FACE_OUTER_BOUND ( 'NONE', #53242, .T. ) ;
#67622=LINE ( 'NONE', #11770, #25810 ) ;
#67659=B_SPLINE_SURFACE_WITH_KNOTS ( 'NONE', 1, 1, ( 
 ( #67530, #26643 ),
 ( #46624, #4863 ) ),
 .UNSPECIFIED., .F., .F., .F.,
 ( 2, 2 ),
 ( 2, 2 ),
 ( 0.000000000000000000, 1.000000000000000000 ),
 ( 0.000000000000000000, 1.000000000000000000 ),
 .UNSPECIFIED. ) ;
#67662=CARTESIAN_POINT ( 'NONE',  ( 0.000000000000000000, 101.5999999999999943, 0.000000000000000000 ) ) ;
#67679=ORIENTED_EDGE ( 'NONE', *, *, #66155, .T. ) ;
#67692=ORIENTED_EDGE ( 'NONE', *, *, #46250, .F. ) ;
#67699=DIRECTION ( 'NONE',  ( 0.000000000000000000, 0.000000000000000000, 1.000000000000000000 ) ) ;
#67741=DIRECTION ( 'NONE',  ( -1.000000000000000000, 0.000000000000000000, 0.000000000000000000 ) ) ;
#67757=CARTESIAN_POINT ( 'NONE',  ( -544.5124999999999318, 53.97500000000000142, 12.69999999999999929 ) ) ;
#67769=CONICAL_SURFACE ( 'NONE', #80885, 39.10000000000005116, 0.7853981633974587151 ) ;
#67772=ORIENTED_EDGE ( 'NONE', *, *, #38639, .F. ) ;
#67774=CARTESIAN_POINT ( 'NONE',  ( -21.42842094847161860, 65.59999999999998010, 41.97446389704171565 ) ) ;
#67817=DIRECTION ( 'NONE',  ( 0.000000000000000000, -1.000000000000000000, -2.913971193241881161E-15 ) ) ;
#67823=ORIENTED_EDGE ( 'NONE', *, *, #87592, .T. ) ;
#67831=CARTESIAN_POINT ( 'NONE',  ( 70.63919639214310564, 100.5999999999999659, 95.21359708083839735 ) ) ;
#67868=VERTEX_POINT ( 'NONE', #56780 ) ;
#67875=VECTOR ( 'NONE', #75970, 1000.000000000000000 ) ;
#67886=LINE ( 'NONE', #60154, #76528 ) ;
#67912=VECTOR ( 'NONE', #17694, 1000.000000000000114 ) ;
#67922=ORIENTED_EDGE ( 'NONE', *, *, #41452, .F. ) ;
#67923=CIRCLE ( 'NONE', #41776, 38.10000000000000142 ) ;
#67924=CARTESIAN_POINT ( 'NONE',  ( -487.2989999999999782, 21.43125000000035030, 6.988054014476359654 ) ) ;
#67986=ADVANCED_FACE ( 'NONE', ( #27394 ), #61908, .F. ) ;
#68038=EDGE_CURVE ( 'NONE', #81729, #23402, #11300, .T. ) ;
#68042=FACE_OUTER_BOUND ( 'NONE', #10862, .T. ) ;
#68100=VECTOR ( 'NONE', #22935, 999.9999999999998863 ) ;
#68106=EDGE_LOOP ( 'NONE', ( #85078, #54883, #68947 ) ) ;
#68128=ORIENTED_EDGE ( 'NONE', *, *, #3169, .F. ) ;
#68160=EDGE_CURVE ( 'NONE', #78132, #41012, #79938, .T. ) ;
#68198=DIRECTION ( 'NONE',  ( -0.6253590364320038564, 0.4667463455728951827, -0.6253590364320190664 ) ) ;
#68211=DIRECTION ( 'NONE',  ( 0.000000000000000000, 0.000000000000000000, 1.000000000000000000 ) ) ;
#68214=CARTESIAN_POINT ( 'NONE',  ( 1.232595164407830946E-29, 69.95000000000000284, 118.3560000000000088 ) ) ;
#68215=ORIENTED_EDGE ( 'NONE', *, *, #35140, .F. ) ;
#68225=LINE ( 'NONE', #6006, #70307 ) ;
#68328=CARTESIAN_POINT ( 'NONE',  ( 0.000000000000000000, 101.5999999999999943, 89.89999999999997726 ) ) ;
#68329=CARTESIAN_POINT ( 'NONE',  ( -254.0000000000000000, 3.174999999999999822, 142.8750000000000000 ) ) ;
#68349=CARTESIAN_POINT ( 'NONE',  ( 61.00843881761244347, 49.07499999999999574, -33.74458626278666884 ) ) ;
#68375=CARTESIAN_POINT ( 'NONE',  ( -487.2989999999999782, 10.16305401447645984, 83.34375000000000000 ) ) ;
#68388=DIRECTION ( 'NONE',  ( 0.8660254037844311581, -0.5000000000000132117, 0.000000000000000000 ) ) ;
#68403=B_SPLINE_SURFACE_WITH_KNOTS ( 'NONE', 1, 1, ( 
 ( #31452, #17395 ),
 ( #23343, #85566 ) ),
 .UNSPECIFIED., .F., .F., .F.,
 ( 2, 2 ),
 ( 2, 2 ),
 ( 0.000000000000000000, 1.000000000000000000 ),
 ( 0.000000000000000000, 1.000000000000000000 ),
 .UNSPECIFIED. ) ;
#68407=DIRECTION ( 'NONE',  ( -1.000000000000000000, 0.000000000000000000, 0.000000000000000000 ) ) ;
#68480=AXIS2_PLACEMENT_3D ( 'NONE', #53952, #5391, #18563 ) ;
#68493=EDGE_CURVE ( 'NONE', #49775, #74329, #5691, .T. ) ;
#68532=CARTESIAN_POINT ( 'NONE',  ( -446.0240000000000009, 104.7749999999999915, 101.5999999999999943 ) ) ;
#68539=CARTESIAN_POINT ( 'NONE',  ( -462.0260000000000105, 53.97500000000000142, -2.412999999999919876 ) ) ;
#68558=CARTESIAN_POINT ( 'NONE',  ( -487.2989999999999782, 93.66249999999999432, 98.73639197104678544 ) ) ;
#68576=ADVANCED_FACE ( 'NONE', ( #76510 ), #7471, .F. ) ;
#68577=DIRECTION ( 'NONE',  ( 0.000000000000000000, 1.000000000000000000, 0.000000000000000000 ) ) ;
#68601=CARTESIAN_POINT ( 'NONE',  ( -492.0614999999999668, 93.66249999999999432, 95.25000000000000000 ) ) ;
#68631=AXIS2_PLACEMENT_3D ( 'NONE', #68558, #89454, #32684 ) ;
#68645=DIRECTION ( 'NONE',  ( 0.000000000000000000, 0.7071067811865426878, 0.7071067811865524577 ) ) ;
#68668=DIRECTION ( 'NONE',  ( 1.821299053822143307E-16, 0.000000000000000000, -1.000000000000000000 ) ) ;
#68709=CARTESIAN_POINT ( 'NONE',  ( -215.9000000000000057, 53.97500000000000142, 50.79999999999999716 ) ) ;
#68714=CARTESIAN_POINT ( 'NONE',  ( -6.657255383333532173, 93.25572935329275026, 118.1691278487518986 ) ) ;
#68749=VECTOR ( 'NONE', #19537, 1000.000000000000000 ) ;
#68767=CARTESIAN_POINT ( 'NONE',  ( -479.3614999999999782, 3.174999999999999822, 101.5999999999999943 ) ) ;
#68768=DIRECTION ( 'NONE',  ( 0.000000000000000000, 0.000000000000000000, -1.000000000000000000 ) ) ;
#68769=FACE_OUTER_BOUND ( 'NONE', #71778, .T. ) ;
#68772=EDGE_CURVE ( 'NONE', #80177, #13052, #86853, .T. ) ;
#68800=CARTESIAN_POINT ( 'NONE',  ( -41.60202597009397607, 65.59999999999998010, 50.85338361873603219 ) ) ;
#68812=ORIENTED_EDGE ( 'NONE', *, *, #74202, .T. ) ;
#68815=PLANE ( 'NONE',  #36004 ) ;
#68826=EDGE_LOOP ( 'NONE', ( #34926, #52680, #88022, #35906 ) ) ;
#68870=ORIENTED_EDGE ( 'NONE', *, *, #17514, .F. ) ;
#68872=ADVANCED_FACE ( 'NONE', ( #57849 ), #85585, .F. ) ;
#68908=ORIENTED_EDGE ( 'NONE', *, *, #66155, .F. ) ;
#68910=DIRECTION ( 'NONE',  ( 0.000000000000000000, -1.000000000000000000, 0.000000000000000000 ) ) ;
#68928=FACE_OUTER_BOUND ( 'NONE', #566, .T. ) ;
#68947=ORIENTED_EDGE ( 'NONE', *, *, #10088, .F. ) ;
#68949=AXIS2_PLACEMENT_3D ( 'NONE', #60473, #25976, #68211 ) ;
#68980=CARTESIAN_POINT ( 'NONE',  ( -462.0260000000000105, 53.97500000000000142, -3.174999999999999822 ) ) ;
#68993=ORIENTED_EDGE ( 'NONE', *, *, #71559, .T. ) ;
#69011=VECTOR ( 'NONE', #51341, 1000.000000000000000 ) ;
#69019=CARTESIAN_POINT ( 'NONE',  ( 50.36513554127332526, 91.40845232887433269, -72.85198609231717626 ) ) ;
#69060=LINE ( 'NONE', #76319, #60235 ) ;
#69070=VECTOR ( 'NONE', #9074, 1000.000000000000000 ) ;
#69079=ORIENTED_EDGE ( 'NONE', *, *, #29712, .T. ) ;
#69085=DIRECTION ( 'NONE',  ( -1.000000000000000000, 0.000000000000000000, 0.000000000000000000 ) ) ;
#69100=VERTEX_POINT ( 'NONE', #85364 ) ;
#69144=DIRECTION ( 'NONE',  ( 0.000000000000000000, 1.000000000000000000, 0.000000000000000000 ) ) ;
#69147=DIRECTION ( 'NONE',  ( -0.000000000000000000, -1.000000000000000000, -0.000000000000000000 ) ) ;
#69187=DIRECTION ( 'NONE',  ( -1.000000000000000000, 7.570719237730541270E-15, 0.000000000000000000 ) ) ;
#69247=ORIENTED_EDGE ( 'NONE', *, *, #3450, .F. ) ;
#69266=AXIS2_PLACEMENT_3D ( 'NONE', #33241, #65, #54991 ) ;
#69310=VECTOR ( 'NONE', #19286, 1000.000000000000114 ) ;
#69311=CARTESIAN_POINT ( 'NONE',  ( -446.0240000000000009, 3.174999999999999822, -1.387778780781445991E-14 ) ) ;
#69319=CARTESIAN_POINT ( 'NONE',  ( 0.000000000000000000, 65.60000000000000853, 0.000000000000000000 ) ) ;
#69321=ORIENTED_EDGE ( 'NONE', *, *, #32572, .F. ) ;
#69358=ORIENTED_EDGE ( 'NONE', *, *, #17792, .F. ) ;
#69362=ADVANCED_FACE ( 'NONE', ( #88923 ), #54355, .F. ) ;
#69364=FACE_OUTER_BOUND ( 'NONE', #84831, .T. ) ;
#69413=AXIS2_PLACEMENT_3D ( 'NONE', #75005, #68198, #61364 ) ;
#69428=ORIENTED_EDGE ( 'NONE', *, *, #40043, .T. ) ;
#69429=AXIS2_PLACEMENT_3D ( 'NONE', #70302, #76676, #64832 ) ;
#69430=CARTESIAN_POINT ( 'NONE',  ( -254.0000000000000000, 3.174999999999999822, -41.27499999999999858 ) ) ;
#69464=CARTESIAN_POINT ( 'NONE',  ( -12.70000000000000107, 82.54999999999999716, 92.46299999999996544 ) ) ;
#69472=CARTESIAN_POINT ( 'NONE',  ( -76.77511553011653689, 55.83576417482189669, 30.88625753091331561 ) ) ;
#69500=AXIS2_PLACEMENT_3D ( 'NONE', #56618, #13949, #36189 ) ;
#69525=ORIENTED_EDGE ( 'NONE', *, *, #17792, .T. ) ;
#69541=CARTESIAN_POINT ( 'NONE',  ( -48.02966122971775320, 91.07499999999996021, -8.747637655308301746E-15 ) ) ;
#69542=EDGE_LOOP ( 'NONE', ( #78821, #17075, #15842, #69525 ) ) ;
#69559=DIRECTION ( 'NONE',  ( 0.000000000000000000, 0.000000000000000000, -1.000000000000000000 ) ) ;
#69570=CARTESIAN_POINT ( 'NONE',  ( -487.2989999999999782, 93.66249999999999432, 98.73639197104678544 ) ) ;
#69617=CARTESIAN_POINT ( 'NONE',  ( -479.3614999999999782, 21.43125000000035030, 6.988054014476359654 ) ) ;
#69622=FACE_OUTER_BOUND ( 'NONE', #27712, .T. ) ;
#69641=CARTESIAN_POINT ( 'NONE',  ( -479.3614999999999782, 10.16305401447644030, 97.63125000000000853 ) ) ;
#69643=CARTESIAN_POINT ( 'NONE',  ( -487.2989999999999782, 7.143750000000339995, 6.988054014476278830 ) ) ;
#69674=ADVANCED_FACE ( 'NONE', ( #72933 ), #31153, .F. ) ;
#69684=CARTESIAN_POINT ( 'NONE',  ( -30.89999999999999858, 53.97499999999997300, 60.80000000000001137 ) ) ;
#69731=ADVANCED_FACE ( 'NONE', ( #60638 ), #68815, .T. ) ;
#69733=LINE ( 'NONE', #25354, #86066 ) ;
#69768=CYLINDRICAL_SURFACE ( 'NONE', #71296, 118.3560000000000088 ) ;
#69777=ORIENTED_EDGE ( 'NONE', *, *, #37622, .T. ) ;
#69778=CARTESIAN_POINT ( 'NONE',  ( -40.89999999999999858, 53.97500000000000142, 50.79999999999999716 ) ) ;
#69791=ADVANCED_FACE ( 'NONE', ( #21573 ), #36085, .F. ) ;
#69808=EDGE_CURVE ( 'NONE', #59384, #62421, #76978, .T. ) ;
#69825=CARTESIAN_POINT ( 'NONE',  ( -55.92138610381699948, 55.69374223142005320, 70.72646601424236223 ) ) ;
#69839=EDGE_CURVE ( 'NONE', #88397, #75550, #44680, .T. ) ;
#69861=EDGE_LOOP ( 'NONE', ( #31425, #8676, #61614, #26480, #43457, #11785, #38066, #73168, #43098, #16703, #71265, #54525, #19452, #66747, #85621, #82930 ) ) ;
#69879=ORIENTED_EDGE ( 'NONE', *, *, #14957, .F. ) ;
#69901=CARTESIAN_POINT ( 'NONE',  ( -479.3614999999999782, 86.51875000000001137, 94.61194598552339130 ) ) ;
#69905=DIRECTION ( 'NONE',  ( -1.000000000000000000, 0.000000000000000000, 0.000000000000000000 ) ) ;
#69910=AXIS2_PLACEMENT_3D ( 'NONE', #84653, #48742, #49647 ) ;
#69914=PRESENTATION_STYLE_ASSIGNMENT (( #14954 ) ) ;
#69915=CYLINDRICAL_SURFACE ( 'NONE', #47709, 4.762500000000001066 ) ;
#69970=CARTESIAN_POINT ( 'NONE',  ( 12.37510959950097877, 79.66588461411475919, 117.9083898578959833 ) ) ;
#69988=ORIENTED_EDGE ( 'NONE', *, *, #73501, .F. ) ;
#70036=CONICAL_SURFACE ( 'NONE', #4733, 89.90000000000000568, 0.7853981633974206344 ) ;
#70046=CARTESIAN_POINT ( 'NONE',  ( 4.059057582146186505, 94.50683581605682093, 118.2888403985303256 ) ) ;
#70052=DIRECTION ( 'NONE',  ( 0.000000000000000000, 0.000000000000000000, -1.000000000000000000 ) ) ;
#70054=CARTESIAN_POINT ( 'NONE',  ( 12.17631217095389573, 79.28385973135301867, 117.7280539260733008 ) ) ;
#70099=DIRECTION ( 'NONE',  ( 0.000000000000000000, 0.000000000000000000, 1.000000000000000000 ) ) ;
#70101=VECTOR ( 'NONE', #67297, 1000.000000000000000 ) ;
#70123=EDGE_CURVE ( 'NONE', #36708, #877, #78230, .T. ) ;
#70130=EDGE_CURVE ( 'NONE', #56709, #22947, #58204, .T. ) ;
#70154=DIRECTION ( 'NONE',  ( -0.000000000000000000, 1.000000000000000000, -0.000000000000000000 ) ) ;
#70166=CARTESIAN_POINT ( 'NONE',  ( 70.63919639214310564, 49.07499999999999574, -53.97512327982435210 ) ) ;
#70168=ORIENTED_EDGE ( 'NONE', *, *, #78019, .T. ) ;
#70213=FACE_OUTER_BOUND ( 'NONE', #3913, .T. ) ;
#70221=ORIENTED_EDGE ( 'NONE', *, *, #813, .T. ) ;
#70253=CARTESIAN_POINT ( 'NONE',  ( -48.02966122971775320, 91.07499999999996021, -8.747637655308301746E-15 ) ) ;
#70260=AXIS2_PLACEMENT_3D ( 'NONE', #5301, #26628, #48387 ) ;
#70267=CARTESIAN_POINT ( 'NONE',  ( -55.84590893209900031, 55.42534759972548386, 70.74779723465208292 ) ) ;
#70275=ORIENTED_EDGE ( 'NONE', *, *, #3146, .T. ) ;
#70278=VECTOR ( 'NONE', #87391, 1000.000000000000000 ) ;
#70300=EDGE_CURVE ( 'NONE', #34776, #16780, #45882, .T. ) ;
#70302=CARTESIAN_POINT ( 'NONE',  ( 0.000000000000000000, -245.0000000000000000, 142.8750000000000000 ) ) ;
#70307=VECTOR ( 'NONE', #61389, 1000.000000000000000 ) ;
#70364=CARTESIAN_POINT ( 'NONE',  ( -76.20994146752570941, 54.60582892396201515, 30.80975041202057341 ) ) ;
#70365=ORIENTED_EDGE ( 'NONE', *, *, #22132, .F. ) ;
#70418=CARTESIAN_POINT ( 'NONE',  ( -215.9000000000000057, 3.174999999999999822, 142.8750000000000000 ) ) ;
#70421=EDGE_CURVE ( 'NONE', #82662, #83342, #900, .T. ) ;
#70437=CARTESIAN_POINT ( 'NONE',  ( -479.3614999999999782, 104.7749999999999915, -1.387778780781445991E-14 ) ) ;
#70443=CARTESIAN_POINT ( 'NONE',  ( -215.9000000000000057, 104.7749999999999915, 142.8750000000000000 ) ) ;
#70455=DIRECTION ( 'NONE',  ( 1.000000000000000000, 0.000000000000000000, 0.000000000000000000 ) ) ;
#70462=FACE_OUTER_BOUND ( 'NONE', #49426, .T. ) ;
#70526=FACE_OUTER_BOUND ( 'NONE', #79746, .T. ) ;
#70533=AXIS2_PLACEMENT_3D ( 'NONE', #67662, #6326, #13152 ) ;
#70542=CARTESIAN_POINT ( 'NONE',  ( -479.3614999999999782, 89.53805401447691281, 18.25625000000039933 ) ) ;
#70548=VERTEX_POINT ( 'NONE', #16323 ) ;
#70563=ORIENTED_EDGE ( 'NONE', *, *, #72659, .T. ) ;
#70570=CARTESIAN_POINT ( 'NONE',  ( -479.3614999999999782, 93.66249999999999432, 82.23860802895320887 ) ) ;
#70674=ORIENTED_EDGE ( 'NONE', *, *, #35821, .T. ) ;
#70703=VECTOR ( 'NONE', #49538, 1000.000000000000114 ) ;
#70717=CARTESIAN_POINT ( 'NONE',  ( -1.663375835020804772, 69.95244002925302595, 118.5450630894975603 ) ) ;
#70731=ORIENTED_EDGE ( 'NONE', *, *, #65446, .F. ) ;
#70745=EDGE_CURVE ( 'NONE', #31377, #34776, #29737, .T. ) ;
#70754=LINE ( 'NONE', #63936, #19008 ) ;
#70765=FACE_BOUND ( 'NONE', #57746, .T. ) ;
#70792=AXIS2_PLACEMENT_3D ( 'NONE', #69311, #7084, #44592 ) ;
#70796=ORIENTED_EDGE ( 'NONE', *, *, #20308, .F. ) ;
#70805=DIRECTION ( 'NONE',  ( 0.000000000000000000, 7.536132396315209176E-17, -1.000000000000000000 ) ) ;
#70819=CARTESIAN_POINT ( 'NONE',  ( 50.42303506447345285, 91.07499999999996021, -73.21698938693724301 ) ) ;
#70820=LINE ( 'NONE', #71712, #1045 ) ;
#70821=ADVANCED_FACE ( 'NONE', ( #50154 ), #28841, .T. ) ;
#70822=ORIENTED_EDGE ( 'NONE', *, *, #30326, .T. ) ;
#70868=CARTESIAN_POINT ( 'NONE',  ( -41.60202597009397607, 40.59999999999997300, 47.03909206933071374 ) ) ;
#70892=ORIENTED_EDGE ( 'NONE', *, *, #53404, .F. ) ;
#70911=CARTESIAN_POINT ( 'NONE',  ( -10.00862986831341317, 74.85114111836281836, 117.9329634167659293 ) ) ;
#70918=VECTOR ( 'NONE', #54312, 1000.000000000000000 ) ;
#70946=LINE ( 'NONE', #82788, #66134 ) ;
#70955=CARTESIAN_POINT ( 'NONE',  ( 11.30434615783713248, 88.13056155020463223, 117.8150791733652341 ) ) ;
#70959=VECTOR ( 'NONE', #48280, 1000.000000000000000 ) ;
#71012=CARTESIAN_POINT ( 'NONE',  ( -446.0240000000000009, 3.174999999999999822, 101.5999999999999943 ) ) ;
#71013=CARTESIAN_POINT ( 'NONE',  ( 0.000000000000000000, 100.5999999999999659, 0.000000000000000000 ) ) ;
#71014=DIRECTION ( 'NONE',  ( 0.5000000000000061062, 0.8660254037844351549, 0.000000000000000000 ) ) ;
#71015=PLANE ( 'NONE',  #55863 ) ;
#71031=EDGE_CURVE ( 'NONE', #53045, #35189, #28886, .T. ) ;
#71038=VERTEX_POINT ( 'NONE', #47352 ) ;
#71056=AXIS2_PLACEMENT_3D ( 'NONE', #61400, #75045, #73701 ) ;
#71064=DIRECTION ( 'NONE',  ( 0.000000000000000000, 0.000000000000000000, -1.000000000000000000 ) ) ;
#71096=CIRCLE ( 'NONE', #59445, 50.79999999999999716 ) ;
#71107=CARTESIAN_POINT ( 'NONE',  ( -240.5296158183964792, 93.66249999999999432, 11.11250000000040217 ) ) ;
#71111=VERTEX_POINT ( 'NONE', #21014 ) ;
#71127=DIRECTION ( 'NONE',  ( 1.000000000000000000, 0.000000000000000000, 0.000000000000000000 ) ) ;
#71156=AXIS2_PLACEMENT_3D ( 'NONE', #79185, #37834, #38265 ) ;
#71171=EDGE_CURVE ( 'NONE', #47557, #42953, #29178, .T. ) ;
#71179=CARTESIAN_POINT ( 'NONE',  ( -55.41748140693382396, 54.70421759738486855, 70.78752196261643803 ) ) ;
#71182=VECTOR ( 'NONE', #43563, 1000.000000000000000 ) ;
#71265=ORIENTED_EDGE ( 'NONE', *, *, #38112, .T. ) ;
#71286=LINE ( 'NONE', #23584, #83892 ) ;
#71296=AXIS2_PLACEMENT_3D ( 'NONE', #69319, #35683, #49750 ) ;
#71301=CARTESIAN_POINT ( 'NONE',  ( -492.0614999999999668, 93.66249999999999432, 90.48749999999999716 ) ) ;
#71310=ORIENTED_EDGE ( 'NONE', *, *, #64656, .F. ) ;
#71311=EDGE_CURVE ( 'NONE', #84869, #33481, #5500, .T. ) ;
#71326=DIRECTION ( 'NONE',  ( 1.000000000000000000, 0.000000000000000000, 0.000000000000000000 ) ) ;
#71399=CARTESIAN_POINT ( 'NONE',  ( 12.60000000000000142, 82.54999999999999716, 92.46299999999996544 ) ) ;
#71418=ORIENTED_EDGE ( 'NONE', *, *, #59325, .T. ) ;
#71420=DIRECTION ( 'NONE',  ( -0.000000000000000000, -0.000000000000000000, 1.000000000000000000 ) ) ;
#71431=B_SPLINE_CURVE_WITH_KNOTS ( 'NONE', 3,
 ( #50400, #15463, #43134, #69970, #84957, #64053, #7738, #56309, #1831, #48593, #473, #22723, #57213, #21371, #28168, #41338, #6837, #28624, #49046, #55855, #63146, #34540, #62243, #30, #84055 ),
 .UNSPECIFIED., .F., .F.,
 ( 4, 2, 2, 2, 2, 2, 2, 2, 2, 1, 2, 2, 4 ),
 ( 0.000000000000000000, 0.002483981393139995941, 0.003725972089710014295, 0.004967962786280032648, 0.007451944179420071090, 0.008693934875990107225, 0.009935925572560145094, 0.01241990696570024859, 0.01366189766227030901, 0.01490388835884037290, 0.01614587905541043159, 0.01738786975198049548, 0.01987185114512061979 ),
 .UNSPECIFIED. ) ;
#71445=EDGE_CURVE ( 'NONE', #24211, #83168, #43385, .T. ) ;
#71460=DIRECTION ( 'NONE',  ( 0.000000000000000000, 6.982966722218760189E-15, -1.000000000000000000 ) ) ;
#71486=ORIENTED_EDGE ( 'NONE', *, *, #83663, .T. ) ;
#71493=EDGE_CURVE ( 'NONE', #7158, #72087, #77674, .T. ) ;
#71516=DIRECTION ( 'NONE',  ( 1.000000000000000000, 0.000000000000000000, 0.000000000000000000 ) ) ;
#71529=EDGE_LOOP ( 'NONE', ( #87051, #67823, #42993, #8364 ) ) ;
#71535=ORIENTED_EDGE ( 'NONE', *, *, #20206, .F. ) ;
#71556=EDGE_LOOP ( 'NONE', ( #33914, #59064, #36385, #89801 ) ) ;
#71558=ORIENTED_EDGE ( 'NONE', *, *, #64149, .F. ) ;
#71559=EDGE_CURVE ( 'NONE', #40087, #74344, #37677, .T. ) ;
#71573=AXIS2_PLACEMENT_3D ( 'NONE', #33708, #82326, #50456 ) ;
#71574=CYLINDRICAL_SURFACE ( 'NONE', #84902, 50.79999999999999716 ) ;
#71579=DIRECTION ( 'NONE',  ( 1.000000000000000000, 0.000000000000000000, 0.000000000000000000 ) ) ;
#71583=FACE_OUTER_BOUND ( 'NONE', #6260, .T. ) ;
#71629=AXIS2_PLACEMENT_3D ( 'NONE', #33444, #54753, #19821 ) ;
#71672=CARTESIAN_POINT ( 'NONE',  ( -469.3583484187089994, 53.97500000000000142, 3.174999999999999822 ) ) ;
#71675=DIRECTION ( 'NONE',  ( 0.000000000000000000, 0.000000000000000000, -1.000000000000000000 ) ) ;
#71676=DIRECTION ( 'NONE',  ( 0.000000000000000000, 0.000000000000000000, -1.000000000000000000 ) ) ;
#71689=AXIS2_PLACEMENT_3D ( 'NONE', #51986, #86106, #65641 ) ;
#71712=CARTESIAN_POINT ( 'NONE',  ( -487.2989999999999782, 93.66249999999999432, 82.23860802895320887 ) ) ;
#71778=EDGE_LOOP ( 'NONE', ( #43290, #88848, #50305, #46361 ) ) ;
#71797=CARTESIAN_POINT ( 'NONE',  ( -12.60000000000000142, 82.54999999999999716, 117.6834004267381744 ) ) ;
#71840=CARTESIAN_POINT ( 'NONE',  ( 11.00055736134227757, 88.91004291464058440, 118.0447018028153394 ) ) ;
#71894=VERTEX_POINT ( 'NONE', #51060 ) ;
#71899=AXIS2_PLACEMENT_3D ( 'NONE', #43731, #51431, #72791 ) ;
#71917=FACE_OUTER_BOUND ( 'NONE', #79822, .T. ) ;
#71958=CONICAL_SURFACE ( 'NONE', #77787, 16.33514202138212923, 0.7853981633974482790 ) ;
#71966=ORIENTED_EDGE ( 'NONE', *, *, #18510, .T. ) ;
#71979=VERTEX_POINT ( 'NONE', #60091 ) ;
#72006=PLANE ( 'NONE',  #17387 ) ;
#72007=LINE ( 'NONE', #3404, #13710 ) ;
#72022=DIRECTION ( 'NONE',  ( 0.2884130866282236250, 0.7071067811865507924, -0.6456143519637524975 ) ) ;
#72048=CARTESIAN_POINT ( 'NONE',  ( -21.42842094847162926, 53.97499999999997300, 41.97446389704172987 ) ) ;
#72072=DIRECTION ( 'NONE',  ( -0.9130365726098600421, 0.000000000000000000, -0.4078776986755215939 ) ) ;
#72087=VERTEX_POINT ( 'NONE', #59649 ) ;
#72095=DIRECTION ( 'NONE',  ( 0.000000000000000000, 1.000000000000000000, 0.000000000000000000 ) ) ;
#72100=VERTEX_POINT ( 'NONE', #3812 ) ;
#72102=FACE_OUTER_BOUND ( 'NONE', #79409, .T. ) ;
#72131=ADVANCED_FACE ( 'NONE', ( #69622 ), #52182, .T. ) ;
#72160=VERTEX_POINT ( 'NONE', #13316 ) ;
#72169=ADVANCED_FACE ( 'NONE', ( #40562 ), #6941, .T. ) ;
#72176=ORIENTED_EDGE ( 'NONE', *, *, #25532, .F. ) ;
#72183=DIRECTION ( 'NONE',  ( 1.000000000000000000, 0.000000000000000000, 0.000000000000000000 ) ) ;
#72185=DIRECTION ( 'NONE',  ( 0.000000000000000000, 0.000000000000000000, 1.000000000000000000 ) ) ;
#72213=DIRECTION ( 'NONE',  ( 0.000000000000000000, -0.8660254037844387076, -0.4999999999999998890 ) ) ;
#72247=LINE ( 'NONE', #79071, #34201 ) ;
#72265=LINE ( 'NONE', #30918, #69011 ) ;
#72298=CARTESIAN_POINT ( 'NONE',  ( 4.446183819022752282, 70.75330535436950186, 118.2730736275787251 ) ) ;
#72339=UNCERTAINTY_MEASURE_WITH_UNIT (LENGTH_MEASURE( 1.000000000000000082E-05 ), #81063, 'distance_accuracy_value', 'NONE');
#72423=ORIENTED_EDGE ( 'NONE', *, *, #14839, .T. ) ;
#72484=CARTESIAN_POINT ( 'NONE',  ( -446.0240000000000009, 14.28750000000026077, 15.87499999999969802 ) ) ;
#72490=EDGE_LOOP ( 'NONE', ( #69777, #79733, #3429, #64700, #38054, #46647 ) ) ;
#72519=AXIS2_PLACEMENT_3D ( 'NONE', #4604, #73635, #39559 ) ;
#72546=VERTEX_POINT ( 'NONE', #18225 ) ;
#72568=ADVANCED_FACE ( 'NONE', ( #65917 ), #17342, .F. ) ;
#72598=EDGE_CURVE ( 'NONE', #35866, #71111, #63902, .T. ) ;
#72650=ORIENTED_EDGE ( 'NONE', *, *, #71031, .F. ) ;
#72659=EDGE_CURVE ( 'NONE', #74753, #81257, #88593, .T. ) ;
#72691=LINE ( 'NONE', #9125, #78585 ) ;
#72692=CARTESIAN_POINT ( 'NONE',  ( -30.89999999999999858, 53.97500000000000142, 40.80000000000000426 ) ) ;
#72693=ORIENTED_EDGE ( 'NONE', *, *, #17959, .F. ) ;
#72701=CARTESIAN_POINT ( 'NONE',  ( -446.0240000000000009, 3.174999999999999822, -1.387778780781445991E-14 ) ) ;
#72704=ORIENTED_EDGE ( 'NONE', *, *, #8697, .T. ) ;
#72728=CARTESIAN_POINT ( 'NONE',  ( 4.478078041421492017, 94.44158826854035738, 118.4720215458495147 ) ) ;
#72739=EDGE_CURVE ( 'NONE', #26268, #61703, #10265, .T. ) ;
#72747=CARTESIAN_POINT ( 'NONE',  ( -41.60202597009397607, 65.59999999999998010, 54.66767516814134353 ) ) ;
#72759=DIRECTION ( 'NONE',  ( 0.000000000000000000, 0.000000000000000000, -1.000000000000000000 ) ) ;
#72791=DIRECTION ( 'NONE',  ( 0.000000000000000000, 7.536132396315209176E-17, -1.000000000000000000 ) ) ;
#72800=VERTEX_POINT ( 'NONE', #19566 ) ;
#72826=CARTESIAN_POINT ( 'NONE',  ( -41.60202597009397607, 40.59999999999997300, 54.66767516814134353 ) ) ;
#72827=CARTESIAN_POINT ( 'NONE',  ( -0.8299567123207916008, 69.87023232701913855, 118.5538273271561707 ) ) ;
#72852=ORIENTED_EDGE ( 'NONE', *, *, #55628, .F. ) ;
#72871=ORIENTED_EDGE ( 'NONE', *, *, #29909, .T. ) ;
#72904=FACE_BOUND ( 'NONE', #25370, .T. ) ;
#72907=VERTEX_POINT ( 'NONE', #70418 ) ;
#72923=DIRECTION ( 'NONE',  ( -0.000000000000000000, 1.000000000000000000, -0.000000000000000000 ) ) ;
#72925=LINE ( 'NONE', #72048, #46107 ) ;
#72933=FACE_OUTER_BOUND ( 'NONE', #60727, .T. ) ;
#72944=EDGE_CURVE ( 'NONE', #83829, #15300, #42239, .T. ) ;
#72958=ORIENTED_EDGE ( 'NONE', *, *, #50031, .F. ) ;
#72960=EDGE_CURVE ( 'NONE', #53086, #10966, #21369, .T. ) ;
#72966=CARTESIAN_POINT ( 'NONE',  ( -465.6921742093550165, 47.62500000000000000, -3.174999999999999822 ) ) ;
#72967=LINE ( 'NONE', #23511, #12723 ) ;
#73034=VERTEX_POINT ( 'NONE', #58549 ) ;
#73043=CARTESIAN_POINT ( 'NONE',  ( -11.75180001297214183, 87.41805222750765836, 117.9724353609281593 ) ) ;
#73105=EDGE_CURVE ( 'NONE', #74526, #55378, #5870, .T. ) ;
#73110=EDGE_CURVE ( 'NONE', #47557, #60931, #79859, .T. ) ;
#73111=DIRECTION ( 'NONE',  ( -1.000000000000000000, 0.000000000000000000, 0.000000000000000000 ) ) ;
#73119=DIRECTION ( 'NONE',  ( 1.000000000000000000, 0.000000000000000000, 0.000000000000000000 ) ) ;
#73123=DIRECTION ( 'NONE',  ( -1.000000000000000000, -0.000000000000000000, -0.000000000000000000 ) ) ;
#73125=VECTOR ( 'NONE', #14387, 1000.000000000000000 ) ;
#73150=CARTESIAN_POINT ( 'NONE',  ( -487.2989999999999782, 86.51875000000001137, 94.61194598552339130 ) ) ;
#73159=CARTESIAN_POINT ( 'NONE',  ( 12.61763483057320911, 84.21901225747508590, 117.8827707503577074 ) ) ;
#73168=ORIENTED_EDGE ( 'NONE', *, *, #12658, .F. ) ;
#73190=AXIS2_PLACEMENT_3D ( 'NONE', #27642, #55322, #63052 ) ;
#73202=EDGE_CURVE ( 'NONE', #65108, #78132, #70754, .T. ) ;
#73212=CARTESIAN_POINT ( 'NONE',  ( -46.60773131249376178, 91.07499999999996021, -44.42500552774628630 ) ) ;
#73230=LINE ( 'NONE', #66870, #63554 ) ;
#73255=DIRECTION ( 'NONE',  ( -0.000000000000000000, 1.000000000000000000, -0.000000000000000000 ) ) ;
#73256=CARTESIAN_POINT ( 'NONE',  ( -254.0000000000000000, 93.66249999999999432, 6.350000000000409983 ) ) ;
#73270=ADVANCED_FACE ( 'NONE', ( #29418 ), #56192, .F. ) ;
#73281=EDGE_CURVE ( 'NONE', #2341, #71979, #75559, .T. ) ;
#73303=DIRECTION ( 'NONE',  ( 0.000000000000000000, 0.000000000000000000, -1.000000000000000000 ) ) ;
#73342=CARTESIAN_POINT ( 'NONE',  ( -479.3614999999999782, 3.174999999999999822, -1.387778780781445991E-14 ) ) ;
#73358=CIRCLE ( 'NONE', #2123, 4.762500000000002842 ) ;
#73379=EDGE_CURVE ( 'NONE', #33481, #56709, #59774, .T. ) ;
#73392=ORIENTED_EDGE ( 'NONE', *, *, #48067, .F. ) ;
#73424=FACE_OUTER_BOUND ( 'NONE', #18878, .T. ) ;
#73444=ORIENTED_EDGE ( 'NONE', *, *, #76242, .T. ) ;
#73448=CARTESIAN_POINT ( 'NONE',  ( -48.02966122971774610, 91.07499999999996021, -43.00307561052233751 ) ) ;
#73468=ORIENTED_EDGE ( 'NONE', *, *, #24278, .T. ) ;
#73476=ADVANCED_FACE ( 'NONE', ( #65272 ), #3052, .T. ) ;
#73501=EDGE_CURVE ( 'NONE', #62421, #74897, #32034, .T. ) ;
#73541=CARTESIAN_POINT ( 'NONE',  ( -487.2989999999999782, 101.9113919710471947, 11.11250000000054072 ) ) ;
#73566=EDGE_CURVE ( 'NONE', #59106, #24430, #5280, .T. ) ;
#73568=ORIENTED_EDGE ( 'NONE', *, *, #60600, .F. ) ;
#73635=DIRECTION ( 'NONE',  ( 0.000000000000000000, -0.4999999999999998890, 0.8660254037844387076 ) ) ;
#73684=VECTOR ( 'NONE', #79891, 1000.000000000000000 ) ;
#73701=DIRECTION ( 'NONE',  ( 0.000000000000000000, 0.000000000000000000, -1.000000000000000000 ) ) ;
#73723=ORIENTED_EDGE ( 'NONE', *, *, #20775, .F. ) ;
#73726=CARTESIAN_POINT ( 'NONE',  ( -48.02966122971776741, 93.07500000000001705, 75.53254848357481421 ) ) ;
#73745=AXIS2_PLACEMENT_3D ( 'NONE', #55763, #27195, #55325 ) ;
#73767=CARTESIAN_POINT ( 'NONE',  ( -487.2989999999999782, 21.43125000000035030, 6.988054014476359654 ) ) ;
#73807=CARTESIAN_POINT ( 'NONE',  ( -465.6921742093539933, 60.32499999999999574, 3.174999999999999822 ) ) ;
#73819=EDGE_LOOP ( 'NONE', ( #67922, #72693 ) ) ;
#73824=CARTESIAN_POINT ( 'NONE',  ( -479.3614999999999782, 104.7749999999999915, -1.387778780781445991E-14 ) ) ;
#73839=CARTESIAN_POINT ( 'NONE',  ( -254.0000000000000000, 14.28749999999982201, 85.72499999999999432 ) ) ;
#73840=ORIENTED_EDGE ( 'NONE', *, *, #35071, .F. ) ;
#73851=AXIS2_PLACEMENT_3D ( 'NONE', #47092, #12608, #74830 ) ;
#73872=AXIS2_PLACEMENT_3D ( 'NONE', #49191, #55998, #83297 ) ;
#73884=LINE ( 'NONE', #24408, #29005 ) ;
#73896=CARTESIAN_POINT ( 'NONE',  ( -487.2989999999999782, 10.16305401447644030, 97.63125000000000853 ) ) ;
#73931=DIRECTION ( 'NONE',  ( 1.000000000000000000, 0.000000000000000000, 0.000000000000000000 ) ) ;
#73950=CARTESIAN_POINT ( 'NONE',  ( -12.70000000000000107, 82.54999999999999716, 117.8738102209307641 ) ) ;
#73960=LINE ( 'NONE', #74412, #31422 ) ;
#73981=CIRCLE ( 'NONE', #58034, 17.33514202138210081 ) ;
#74016=PRODUCT_CONTEXT ( 'NONE', #44601, 'mechanical' ) ;
#74055=CARTESIAN_POINT ( 'NONE',  ( -487.2989999999999782, 7.143750000000280487, 15.23694598552305024 ) ) ;
#74056=ORIENTED_EDGE ( 'NONE', *, *, #51290, .T. ) ;
#74058=ORIENTED_EDGE ( 'NONE', *, *, #5522, .F. ) ;
#74071=FACE_OUTER_BOUND ( 'NONE', #24644, .T. ) ;
#74076=AXIS2_PLACEMENT_3D ( 'NONE', #84937, #78574, #23163 ) ;
#74097=ORIENTED_EDGE ( 'NONE', *, *, #22939, .F. ) ;
#74098=DIRECTION ( 'NONE',  ( 1.000000000000000000, 0.000000000000000000, 0.000000000000000000 ) ) ;
#74106=EDGE_CURVE ( 'NONE', #29846, #19430, #15022, .T. ) ;
#74135=ORIENTED_EDGE ( 'NONE', *, *, #64575, .F. ) ;
#74142=LINE ( 'NONE', #11916, #82859 ) ;
#74143=DIRECTION ( 'NONE',  ( 0.5000000000000061062, 0.8660254037844351549, 0.000000000000000000 ) ) ;
#74159=EDGE_LOOP ( 'NONE', ( #74588, #47721, #51746, #27300 ) ) ;
#74180=LINE ( 'NONE', #86924, #56343 ) ;
#74184=CARTESIAN_POINT ( 'NONE',  ( -11.32175285073831894, 88.14108913799663014, 117.8136741508921261 ) ) ;
#74202=EDGE_CURVE ( 'NONE', #67042, #15378, #17699, .T. ) ;
#74236=DIRECTION ( 'NONE',  ( -1.000000000000000000, 7.570719237730541270E-15, 0.000000000000000000 ) ) ;
#74281=CARTESIAN_POINT ( 'NONE',  ( -76.76779673090611311, 55.97500000000000142, 30.90025125786759830 ) ) ;
#74302=PRODUCT_DEFINITION_SHAPE ( 'NONE', 'NONE',  #57145 ) ;
#74329=VERTEX_POINT ( 'NONE', #68532 ) ;
#74344=VERTEX_POINT ( 'NONE', #27636 ) ;
#74346=AXIS2_PLACEMENT_3D ( 'NONE', #52983, #46640, #88907 ) ;
#74361=LINE ( 'NONE', #75261, #21909 ) ;
#74369=FACE_OUTER_BOUND ( 'NONE', #39069, .T. ) ;
#74386=VECTOR ( 'NONE', #47844, 1000.000000000000000 ) ;
#74403=EDGE_CURVE ( 'NONE', #74329, #74526, #25852, .T. ) ;
#74407=EDGE_CURVE ( 'NONE', #26268, #9288, #19934, .T. ) ;
#74412=CARTESIAN_POINT ( 'NONE',  ( -64.09238476222100189, 53.97500000000000142, 58.69734786913941349 ) ) ;
#74415=CARTESIAN_POINT ( 'NONE',  ( 70.63919639214310564, 91.07499999999996021, 53.63573739454427880 ) ) ;
#74420=ORIENTED_EDGE ( 'NONE', *, *, #2165, .T. ) ;
#74421=ORIENTED_EDGE ( 'NONE', *, *, #25265, .T. ) ;
#74435=AXIS2_PLACEMENT_3D ( 'NONE', #25855, #81290, #4961 ) ;
#74449=EDGE_LOOP ( 'NONE', ( #65124, #69079 ) ) ;
#74451=EDGE_LOOP ( 'NONE', ( #35287, #46676, #48451, #68128, #73723 ) ) ;
#74494=VERTEX_POINT ( 'NONE', #20390 ) ;
#74495=ORIENTED_EDGE ( 'NONE', *, *, #87316, .T. ) ;
#74504=CARTESIAN_POINT ( 'NONE',  ( 0.000000000000000000, 100.5999999999999659, 0.000000000000000000 ) ) ;
#74505=CARTESIAN_POINT ( 'NONE',  ( 4.665904304751416087E-15, 65.60000000000000853, -38.10000000000000142 ) ) ;
#74518=CARTESIAN_POINT ( 'NONE',  ( 4.788368984666157546E-15, 92.07499999999998863, -39.10000000000005116 ) ) ;
#74526=VERTEX_POINT ( 'NONE', #2181 ) ;
#74532=CARTESIAN_POINT ( 'NONE',  ( -479.3614999999999782, 104.7749999999999915, -1.387778780781445991E-14 ) ) ;
#74543=ORIENTED_EDGE ( 'NONE', *, *, #64708, .T. ) ;
#74584=ORIENTED_EDGE ( 'NONE', *, *, #75637, .T. ) ;
#74586=ADVANCED_FACE ( 'NONE', ( #36246 ), #8974, .T. ) ;
#74588=ORIENTED_EDGE ( 'NONE', *, *, #59617, .T. ) ;
#74595=EDGE_CURVE ( 'NONE', #47865, #27915, #57573, .T. ) ;
#74599=ORIENTED_EDGE ( 'NONE', *, *, #86162, .T. ) ;
#74620=DIRECTION ( 'NONE',  ( 0.000000000000000000, 0.000000000000000000, 1.000000000000000000 ) ) ;
#74629=ORIENTED_EDGE ( 'NONE', *, *, #8697, .F. ) ;
#74649=VERTEX_POINT ( 'NONE', #28072 ) ;
#74670=FACE_OUTER_BOUND ( 'NONE', #79394, .T. ) ;
#74702=VERTEX_POINT ( 'NONE', #18469 ) ;
#74706=CARTESIAN_POINT ( 'NONE',  ( -47.06748920650090184, 92.32491709964729409, 74.53227049051039899 ) ) ;
#74753=VERTEX_POINT ( 'NONE', #79835 ) ;
#74758=EDGE_LOOP ( 'NONE', ( #61868, #50610, #16657, #86946 ) ) ;
#74771=DIRECTION ( 'NONE',  ( 0.000000000000000000, 0.000000000000000000, -1.000000000000000000 ) ) ;
#74773=VECTOR ( 'NONE', #16305, 1000.000000000000000 ) ;
#74775=CIRCLE ( 'NONE', #58815, 36.57600000000000051 ) ;
#74776=CIRCLE ( 'NONE', #55884, 3.814291549405317117 ) ;
#74786=CARTESIAN_POINT ( 'NONE',  ( -487.2989999999999782, 93.66249999999999432, 6.350000000000409983 ) ) ;
#74791=DIRECTION ( 'NONE',  ( 0.000000000000000000, -1.000000000000000000, 0.000000000000000000 ) ) ;
#74826=ORIENTED_EDGE ( 'NONE', *, *, #2141, .T. ) ;
#74830=DIRECTION ( 'NONE',  ( 0.000000000000000000, 1.000000000000000000, 1.056314557550181068E-14 ) ) ;
#74836=DIRECTION ( 'NONE',  ( 0.000000000000000000, 0.000000000000000000, 1.000000000000000000 ) ) ;
#74861=DIRECTION ( 'NONE',  ( 0.000000000000000000, 0.000000000000000000, 1.000000000000000000 ) ) ;
#74871=FACE_OUTER_BOUND ( 'NONE', #26137, .T. ) ;
#74875=CARTESIAN_POINT ( 'NONE',  ( 0.000000000000000000, 65.60000000000000853, 38.10000000000000142 ) ) ;
#74878=DIRECTION ( 'NONE',  ( -1.000000000000000000, 0.000000000000000000, 0.000000000000000000 ) ) ;
#74897=VERTEX_POINT ( 'NONE', #74786 ) ;
#74902=CARTESIAN_POINT ( 'NONE',  ( -479.3614999999999782, 104.7749999999999915, -1.387778780781445991E-14 ) ) ;
#74911=CARTESIAN_POINT ( 'NONE',  ( -0.8023776826656670025, 53.97499999999997300, -4.197052493943455254 ) ) ;
#74915=CIRCLE ( 'NONE', #37180, 3.814291549405317117 ) ;
#74922=ADVANCED_FACE ( 'NONE', ( #6203 ), #82074, .T. ) ;
#74933=DIRECTION ( 'NONE',  ( 1.000000000000000000, 0.000000000000000000, 0.000000000000000000 ) ) ;
#74988=ORIENTED_EDGE ( 'NONE', *, *, #78941, .T. ) ;
#75005=CARTESIAN_POINT ( 'NONE',  ( -46.60773131249376178, 91.07499999999996021, -44.42500552774628630 ) ) ;
#75021=CARTESIAN_POINT ( 'NONE',  ( 0.000000000000000000, 92.07499999999998863, 0.000000000000000000 ) ) ;
#75045=DIRECTION ( 'NONE',  ( -0.000000000000000000, -1.000000000000000000, -0.000000000000000000 ) ) ;
#75092=ORIENTED_EDGE ( 'NONE', *, *, #39639, .F. ) ;
#75121=CARTESIAN_POINT ( 'NONE',  ( -47.02966122971773189, 92.07499999999998863, -8.565507749926084753E-15 ) ) ;
#75129=ADVANCED_FACE ( 'NONE', ( #56106 ), #50652, .T. ) ;
#75155=EDGE_CURVE ( 'NONE', #87961, #74344, #63397, .T. ) ;
#75163=VERTEX_POINT ( 'NONE', #77476 ) ;
#75170=CARTESIAN_POINT ( 'NONE',  ( -479.3614999999999782, 104.7749999999999915, 101.5999999999999943 ) ) ;
#75183=CARTESIAN_POINT ( 'NONE',  ( 61.00843881761244347, 49.07499999999999574, -53.97512327982435210 ) ) ;
#75204=EDGE_LOOP ( 'NONE', ( #24170, #1116, #22150 ) ) ;
#75239=CYLINDRICAL_SURFACE ( 'NONE', #70260, 4.762500000000002842 ) ;
#75261=CARTESIAN_POINT ( 'NONE',  ( -15.89999999999999680, 53.97500000000000142, 30.79999999999999361 ) ) ;
#75278=EDGE_LOOP ( 'NONE', ( #22390, #57781, #88130, #21443 ) ) ;
#75292=DIRECTION ( 'NONE',  ( -0.000000000000000000, -0.000000000000000000, 1.000000000000000000 ) ) ;
#75314=EDGE_LOOP ( 'NONE', ( #23605, #31879, #73468, #18455, #4140, #74421 ) ) ;
#75325=PLANE ( 'NONE',  #66323 ) ;
#75349=FACE_OUTER_BOUND ( 'NONE', #45014, .T. ) ;
#75390=B_SPLINE_CURVE_WITH_KNOTS ( 'NONE', 3,
 ( #1462, #545, #55937, #28244, #83682, #43666, #70046, #63677, #35504, #63226, #28707, #77760, #15083, #21907, #49575, #56842, #84588, #70955, #8728, #1902, #59518, #30941, #30055, #2801, #36864, #38201 ),
 .UNSPECIFIED., .F., .F.,
 ( 4, 2, 2, 2, 2, 2, 2, 2, 2, 2, 2, 2, 4 ),
 ( 0.01971520310360850431, 0.02094683101846679663, 0.02217845893332509241, 0.02464171476304167704, 0.02587334267789997283, 0.02710497059275826515, 0.02956822642247482896, 0.03203148225219139278, 0.03326311016704969203, 0.03449473808190799129, 0.03695799391162458980, 0.03818962182648288906, 0.03942124974134118831 ),
 .UNSPECIFIED. ) ;
#75396=EDGE_CURVE ( 'NONE', #46111, #296, #25628, .T. ) ;
#75448=ORIENTED_EDGE ( 'NONE', *, *, #75637, .F. ) ;
#75455=LINE ( 'NONE', #49509, #84017 ) ;
#75471=CARTESIAN_POINT ( 'NONE',  ( -487.2989999999999782, 89.53805401447711176, 3.968750000000410338 ) ) ;
#75490=VECTOR ( 'NONE', #50882, 1000.000000000000114 ) ;
#75492=VERTEX_POINT ( 'NONE', #39257 ) ;
#75499=CARTESIAN_POINT ( 'NONE',  ( -31.27367473141074683, 54.97499999999996589, 74.45358409497265484 ) ) ;
#75523=ORIENTED_EDGE ( 'NONE', *, *, #89219, .T. ) ;
#75535=EDGE_CURVE ( 'NONE', #49587, #87146, #54198, .T. ) ;
#75550=VERTEX_POINT ( 'NONE', #26979 ) ;
#75559=CIRCLE ( 'NONE', #36402, 4.762500000000002842 ) ;
#75604=EDGE_CURVE ( 'NONE', #14208, #37970, #59837, .T. ) ;
#75613=CARTESIAN_POINT ( 'NONE',  ( -55.89999999999999858, 55.97500000000000142, 70.79999999999999716 ) ) ;
#75631=LINE ( 'NONE', #88373, #42919 ) ;
#75637=EDGE_CURVE ( 'NONE', #14474, #10702, #86005, .T. ) ;
#75662=VERTEX_POINT ( 'NONE', #20615 ) ;
#75684=CARTESIAN_POINT ( 'NONE',  ( -40.89999999999999858, 53.97500000000000142, 60.79999999999999716 ) ) ;
#75685=DIRECTION ( 'NONE',  ( -0.4999999999999932832, 0.8660254037844424824, 0.000000000000000000 ) ) ;
#75703=FACE_OUTER_BOUND ( 'NONE', #74758, .T. ) ;
#75712=AXIS2_PLACEMENT_3D ( 'NONE', #73342, #51985, #10670 ) ;
#75728=DIRECTION ( 'NONE',  ( 0.000000000000000000, -1.000000000000000000, 0.000000000000000000 ) ) ;
#75764=ORIENTED_EDGE ( 'NONE', *, *, #82516, .F. ) ;
#75778=ORIENTED_EDGE ( 'NONE', *, *, #58636, .T. ) ;
#75785=CARTESIAN_POINT ( 'NONE',  ( 0.000000000000000000, 101.5999999999999943, 0.000000000000000000 ) ) ;
#75855=ADVANCED_FACE ( 'NONE', ( #65954 ), #55540, .T. ) ;
#75915=CYLINDRICAL_SURFACE ( 'NONE', #81138, 88.90000000000000568 ) ;
#75938=EDGE_CURVE ( 'NONE', #85611, #83342, #25522, .T. ) ;
#75958=CYLINDRICAL_SURFACE ( 'NONE', #41706, 38.10000000000000142 ) ;
#75966=ORIENTED_EDGE ( 'NONE', *, *, #36997, .T. ) ;
#75970=DIRECTION ( 'NONE',  ( 0.000000000000000000, 0.4999999999999897304, 0.8660254037844445918 ) ) ;
#75986=ORIENTED_EDGE ( 'NONE', *, *, #62317, .F. ) ;
#76001=ORIENTED_EDGE ( 'NONE', *, *, #76557, .F. ) ;
#76003=EDGE_CURVE ( 'NONE', #43910, #52044, #67171, .T. ) ;
#76011=AXIS2_PLACEMENT_3D ( 'NONE', #75684, #88424, #39792 ) ;
#76013=CARTESIAN_POINT ( 'NONE',  ( -254.0000000000000000, 104.7749999999999915, -41.27499999999999858 ) ) ;
#76032=PLANE ( 'NONE',  #42167 ) ;
#76039=DIRECTION ( 'NONE',  ( 0.9130365726098601531, 0.000000000000000000, 0.4078776986755214828 ) ) ;
#76076=AXIS2_PLACEMENT_3D ( 'NONE', #13158, #74933, #34928 ) ;
#76105=DIRECTION ( 'NONE',  ( 0.000000000000000000, 0.000000000000000000, 1.000000000000000000 ) ) ;
#76110=ORIENTED_EDGE ( 'NONE', *, *, #17093, .T. ) ;
#76113=PLANE ( 'NONE',  #70792 ) ;
#76152=EDGE_LOOP ( 'NONE', ( #25858, #20587, #27835, #26123, #28523, #80703 ) ) ;
#76156=ADVANCED_FACE ( 'NONE', ( #38541, #64919 ), #57646, .T. ) ;
#76168=DIRECTION ( 'NONE',  ( 1.000000000000000000, 0.000000000000000000, 0.000000000000000000 ) ) ;
#76187=VERTEX_POINT ( 'NONE', #49264 ) ;
#76194=CARTESIAN_POINT ( 'NONE',  ( -47.11752803141011015, 100.5999999999999659, 108.7909173056707317 ) ) ;
#76208=ORIENTED_EDGE ( 'NONE', *, *, #78565, .F. ) ;
#76221=CARTESIAN_POINT ( 'NONE',  ( 0.000000000000000000, 65.60000000000000853, 0.000000000000000000 ) ) ;
#76242=EDGE_CURVE ( 'NONE', #1472, #56709, #69733, .T. ) ;
#76246=DIRECTION ( 'NONE',  ( 0.000000000000000000, 0.000000000000000000, 1.000000000000000000 ) ) ;
#76250=AXIS2_PLACEMENT_3D ( 'NONE', #35894, #9541, #49956 ) ;
#76271=FACE_OUTER_BOUND ( 'NONE', #10494, .T. ) ;
#76272=AXIS2_PLACEMENT_3D ( 'NONE', #58301, #49802, #80545 ) ;
#76273=CARTESIAN_POINT ( 'NONE',  ( -240.5296158183964792, 14.28750000000026077, 11.11249999999970051 ) ) ;
#76279=EDGE_CURVE ( 'NONE', #1004, #79764, #53486, .T. ) ;
#76281=CARTESIAN_POINT ( 'NONE',  ( -76.76779673090611311, 55.97500000000000142, 30.90025125786759830 ) ) ;
#76298=EDGE_LOOP ( 'NONE', ( #12687, #60908, #44841, #14031, #40345, #36689 ) ) ;
#76319=CARTESIAN_POINT ( 'NONE',  ( -487.2989999999999782, 10.16305401447645984, 83.34375000000000000 ) ) ;
#76351=FACE_OUTER_BOUND ( 'NONE', #44411, .T. ) ;
#76363=EDGE_CURVE ( 'NONE', #43607, #14882, #7600, .T. ) ;
#76375=CARTESIAN_POINT ( 'NONE',  ( 0.000000000000000000, 82.54999999999999716, 89.46299999999996544 ) ) ;
#76376=DIRECTION ( 'NONE',  ( 0.000000000000000000, 0.5000000000000007772, -0.8660254037844381525 ) ) ;
#76398=LINE ( 'NONE', #7803, #63241 ) ;
#76464=CARTESIAN_POINT ( 'NONE',  ( -17.13243906362141900, 54.97499999999995879, 42.79834678115690849 ) ) ;
#76470=FACE_OUTER_BOUND ( 'NONE', #56676, .T. ) ;
#76493=ORIENTED_EDGE ( 'NONE', *, *, #87131, .F. ) ;
#76510=FACE_OUTER_BOUND ( 'NONE', #80550, .T. ) ;
#76528=VECTOR ( 'NONE', #47871, 999.9999999999998863 ) ;
#76541=DIRECTION ( 'NONE',  ( -0.7071067811865474617, 0.7071067811865474617, 0.000000000000000000 ) ) ;
#76557=EDGE_CURVE ( 'NONE', #51377, #79343, #15348, .T. ) ;
#76586=DIRECTION ( 'NONE',  ( 0.000000000000000000, 1.000000000000000000, 0.000000000000000000 ) ) ;
#76603=ORIENTED_EDGE ( 'NONE', *, *, #46536, .F. ) ;
#76608=ORIENTED_EDGE ( 'NONE', *, *, #58820, .F. ) ;
#76652=LINE ( 'NONE', #28490, #22724 ) ;
#76657=VERTEX_POINT ( 'NONE', #51625 ) ;
#76676=DIRECTION ( 'NONE',  ( -0.000000000000000000, 0.000000000000000000, -1.000000000000000000 ) ) ;
#76687=DIRECTION ( 'NONE',  ( 0.000000000000000000, 0.8660254037844387076, 0.4999999999999998890 ) ) ;
#76689=ADVANCED_FACE ( 'NONE', ( #37575 ), #78480, .T. ) ;
#76709=VERTEX_POINT ( 'NONE', #78920 ) ;
#76725=EDGE_CURVE ( 'NONE', #78995, #19810, #30805, .T. ) ;
#76732=CARTESIAN_POINT ( 'NONE',  ( -76.71224887342795284, 55.42750769018135060, 30.85235132533246372 ) ) ;
#76735=ORIENTED_EDGE ( 'NONE', *, *, #55345, .T. ) ;
#76744=VERTEX_POINT ( 'NONE', #84841 ) ;
#76762=ORIENTED_EDGE ( 'NONE', *, *, #26702, .F. ) ;
#76789=DIRECTION ( 'NONE',  ( -1.000000000000000000, 0.000000000000000000, 0.000000000000000000 ) ) ;
#76800=EDGE_LOOP ( 'NONE', ( #76001, #65370 ) ) ;
#76803=DIRECTION ( 'NONE',  ( -0.000000000000000000, 1.000000000000000000, -0.000000000000000000 ) ) ;
#76813=CARTESIAN_POINT ( 'NONE',  ( -487.2989999999999782, 7.143750000000280487, 15.23694598552305024 ) ) ;
#76830=ORIENTED_EDGE ( 'NONE', *, *, #12658, .T. ) ;
#76841=ORIENTED_EDGE ( 'NONE', *, *, #36867, .F. ) ;
#76853=EDGE_CURVE ( 'NONE', #37391, #86124, #81611, .T. ) ;
#76903=VERTEX_POINT ( 'NONE', #3935 ) ;
#76929=EDGE_LOOP ( 'NONE', ( #22067, #8382, #68215, #59801, #13203 ) ) ;
#76944=CARTESIAN_POINT ( 'NONE',  ( -50.35902679310718355, 64.60000000000000853, 27.95514712793348977 ) ) ;
#76978=LINE ( 'NONE', #56052, #47584 ) ;
#76992=EDGE_LOOP ( 'NONE', ( #28265, #16174, #28447, #69358, #2613 ) ) ;
#77002=ORIENTED_EDGE ( 'NONE', *, *, #46310, .F. ) ;
#77015=FACE_OUTER_BOUND ( 'NONE', #19196, .T. ) ;
#77020=ORIENTED_EDGE ( 'NONE', *, *, #73501, .T. ) ;
#77028=ORIENTED_EDGE ( 'NONE', *, *, #82648, .F. ) ;
#77033=DIRECTION ( 'NONE',  ( 1.821299053822143307E-16, 0.000000000000000000, -1.000000000000000000 ) ) ;
#77071=ADVANCED_FACE ( 'NONE', ( #50636 ), #70036, .F. ) ;
#77082=EDGE_CURVE ( 'NONE', #18243, #88352, #38786, .T. ) ;
#77110=PLANE ( 'NONE',  #63359 ) ;
#77113=ORIENTED_EDGE ( 'NONE', *, *, #21687, .F. ) ;
#77130=DIRECTION ( 'NONE',  ( -1.000000000000000000, 0.000000000000000000, 0.000000000000000000 ) ) ;
#77143=DIRECTION ( 'NONE',  ( 1.000000000000000000, 0.000000000000000000, 0.000000000000000000 ) ) ;
#77145=FACE_OUTER_BOUND ( 'NONE', #23043, .T. ) ;
#77165=CARTESIAN_POINT ( 'NONE',  ( 12.70000000000000107, 82.54999999999999716, 92.46299999999996544 ) ) ;
#77188=CARTESIAN_POINT ( 'NONE',  ( -76.30649458666536589, 54.70491969191439807, 30.81302321914488473 ) ) ;
#77202=VERTEX_POINT ( 'NONE', #88309 ) ;
#77205=ORIENTED_EDGE ( 'NONE', *, *, #83663, .F. ) ;
#77207=VERTEX_POINT ( 'NONE', #88751 ) ;
#77212=LINE ( 'NONE', #20897, #11396 ) ;
#77234=EDGE_LOOP ( 'NONE', ( #36176, #65596 ) ) ;
#77246=CARTESIAN_POINT ( 'NONE',  ( 70.63919639214310564, 100.5999999999999659, 0.000000000000000000 ) ) ;
#77251=ORIENTED_EDGE ( 'NONE', *, *, #34064, .F. ) ;
#77304=CARTESIAN_POINT ( 'NONE',  ( 61.00843881761244347, 49.07499999999999574, -53.97512327982435210 ) ) ;
#77317=CARTESIAN_POINT ( 'NONE',  ( 50.42303506447345285, 91.07499999999996021, -73.21698938693724301 ) ) ;
#77322=EDGE_LOOP ( 'NONE', ( #47679, #53146, #32800, #44779 ) ) ;
#77325=DIRECTION ( 'NONE',  ( -1.000000000000000000, 0.000000000000000000, 0.000000000000000000 ) ) ;
#77332=ORIENTED_EDGE ( 'NONE', *, *, #25532, .T. ) ;
#77347=DIRECTION ( 'NONE',  ( 0.000000000000000000, 1.000000000000000000, 1.047445008332813989E-14 ) ) ;
#77361=LINE ( 'NONE', #76464, #20178 ) ;
#77363=DIRECTION ( 'NONE',  ( 0.000000000000000000, 0.000000000000000000, 1.000000000000000000 ) ) ;
#77424=DIRECTION ( 'NONE',  ( 0.000000000000000000, 0.000000000000000000, 1.000000000000000000 ) ) ;
#77444=EDGE_LOOP ( 'NONE', ( #16736, #44923, #24902, #53883, #76208, #34558, #6388, #78209 ) ) ;
#77452=AXIS2_PLACEMENT_3D ( 'NONE', #85693, #16198, #64783 ) ;
#77476=CARTESIAN_POINT ( 'NONE',  ( -34.93928583487483763, 53.97499999999997300, 35.93880153443800651 ) ) ;
#77505=CARTESIAN_POINT ( 'NONE',  ( -479.3614999999999782, 86.51875000000001137, 86.36305401447658880 ) ) ;
#77513=ORIENTED_EDGE ( 'NONE', *, *, #30932, .T. ) ;
#77530=CARTESIAN_POINT ( 'NONE',  ( -11.57414189257196568, 77.30572722422043341, 117.9897876170239073 ) ) ;
#77547=AXIS2_PLACEMENT_3D ( 'NONE', #59027, #86766, #47182 ) ;
#77549=ORIENTED_EDGE ( 'NONE', *, *, #49985, .T. ) ;
#77562=ORIENTED_EDGE ( 'NONE', *, *, #51455, .F. ) ;
#77564=VERTEX_POINT ( 'NONE', #49618 ) ;
#77575=CIRCLE ( 'NONE', #665, 88.90000000000000568 ) ;
#77609=ORIENTED_EDGE ( 'NONE', *, *, #38923, .T. ) ;
#77616=DIRECTION ( 'NONE',  ( 0.000000000000000000, 0.000000000000000000, 1.000000000000000000 ) ) ;
#77647=ORIENTED_EDGE ( 'NONE', *, *, #79178, .T. ) ;
#77674=LINE ( 'NONE', #70868, #62260 ) ;
#77684=ORIENTED_EDGE ( 'NONE', *, *, #64682, .F. ) ;
#77690=ADVANCED_FACE ( 'NONE', ( #82181 ), #27191, .F. ) ;
#77693=ADVANCED_FACE ( 'NONE', ( #75349 ), #82631, .T. ) ;
#77721=CARTESIAN_POINT ( 'NONE',  ( -8.616376681309702690, 73.34747254003858075, 118.0423040787594005 ) ) ;
#77723=EDGE_CURVE ( 'NONE', #4807, #24603, #28007, .T. ) ;
#77739=ORIENTED_EDGE ( 'NONE', *, *, #4282, .T. ) ;
#77751=FACE_OUTER_BOUND ( 'NONE', #7265, .T. ) ;
#77760=CARTESIAN_POINT ( 'NONE',  ( 7.685743261040695273, 92.56811239613027453, 118.1081662844706557 ) ) ;
#77774=CARTESIAN_POINT ( 'NONE',  ( -3.266173478975160638, 94.72629918563912099, 118.3115834712042584 ) ) ;
#77787=AXIS2_PLACEMENT_3D ( 'NONE', #59235, #25615, #19260 ) ;
#77820=DIRECTION ( 'NONE',  ( 0.000000000000000000, 1.000000000000000000, 0.000000000000000000 ) ) ;
#77829=VERTEX_POINT ( 'NONE', #35786 ) ;
#77842=VERTEX_POINT ( 'NONE', #14010 ) ;
#77900=ORIENTED_EDGE ( 'NONE', *, *, #31846, .T. ) ;
#77914=CYLINDRICAL_SURFACE ( 'NONE', #66021, 4.762500000000001066 ) ;
#77915=ADVANCED_FACE ( 'NONE', ( #35336 ), #63499, .F. ) ;
#77919=VERTEX_POINT ( 'NONE', #7647 ) ;
#77921=VECTOR ( 'NONE', #9267, 1000.000000000000000 ) ;
#77935=CARTESIAN_POINT ( 'NONE',  ( -15.89999999999999680, 53.97500000000000142, 30.79999999999999361 ) ) ;
#77944=FACE_OUTER_BOUND ( 'NONE', #76298, .T. ) ;
#77960=LINE ( 'NONE', #77505, #63261 ) ;
#77968=ORIENTED_EDGE ( 'NONE', *, *, #73202, .F. ) ;
#77995=CARTESIAN_POINT ( 'NONE',  ( -254.0000000000000000, 53.97500000000000142, 50.79999999999999716 ) ) ;
#78019=EDGE_CURVE ( 'NONE', #50313, #54435, #36705, .T. ) ;
#78023=EDGE_CURVE ( 'NONE', #3353, #296, #79837, .T. ) ;
#78024=CARTESIAN_POINT ( 'NONE',  ( -446.0240000000000009, 14.28749999999982201, 90.48749999999999716 ) ) ;
#78081=VECTOR ( 'NONE', #62396, 1000.000000000000000 ) ;
#78132=VERTEX_POINT ( 'NONE', #47054 ) ;
#78144=VERTEX_POINT ( 'NONE', #40706 ) ;
#78154=PLANE ( 'NONE',  #76250 ) ;
#78170=LINE ( 'NONE', #8670, #47597 ) ;
#78178=CIRCLE ( 'NONE', #14354, 20.00000000000000355 ) ;
#78209=ORIENTED_EDGE ( 'NONE', *, *, #75604, .T. ) ;
#78212=DIRECTION ( 'NONE',  ( 0.000000000000000000, 1.000000000000000000, 0.000000000000000000 ) ) ;
#78218=DIRECTION ( 'NONE',  ( 0.000000000000000000, 0.4999999999999998890, -0.8660254037844387076 ) ) ;
#78230=LINE ( 'NONE', #65466, #1204 ) ;
#78254=FACE_OUTER_BOUND ( 'NONE', #45896, .T. ) ;
#78272=AXIS2_PLACEMENT_3D ( 'NONE', #8492, #48435, #49800 ) ;
#78323=LINE ( 'NONE', #85586, #28992 ) ;
#78332=ORIENTED_EDGE ( 'NONE', *, *, #83309, .T. ) ;
#78336=EDGE_CURVE ( 'NONE', #79343, #64560, #42570, .T. ) ;
#78357=AXIS2_PLACEMENT_3D ( 'NONE', #50553, #176, #21533 ) ;
#78379=ORIENTED_EDGE ( 'NONE', *, *, #44343, .T. ) ;
#78397=CARTESIAN_POINT ( 'NONE',  ( -446.0240000000000009, 53.97500000000000142, 50.79999999999999716 ) ) ;
#78408=CIRCLE ( 'NONE', #65280, 3.700000000000001954 ) ;
#78435=CARTESIAN_POINT ( 'NONE',  ( 0.000000000000000000, 101.6000000000000227, 0.000000000000000000 ) ) ;
#78439=VECTOR ( 'NONE', #1829, 1000.000000000000114 ) ;
#78480=CYLINDRICAL_SURFACE ( 'NONE', #24971, 3.700000000000001954 ) ;
#78493=DIRECTION ( 'NONE',  ( 1.821299053822143307E-16, 0.000000000000000000, -1.000000000000000000 ) ) ;
#78517=EDGE_LOOP ( 'NONE', ( #2262, #41608 ) ) ;
#78525=CARTESIAN_POINT ( 'NONE',  ( -458.3598257906459708, 60.32499999999999574, 3.174999999999999822 ) ) ;
#78565=EDGE_CURVE ( 'NONE', #67868, #53581, #84759, .T. ) ;
#78574=DIRECTION ( 'NONE',  ( 0.000000000000000000, -1.000000000000000000, -0.000000000000000000 ) ) ;
#78585=VECTOR ( 'NONE', #10455, 1000.000000000000000 ) ;
#78586=PLANE ( 'NONE',  #56559 ) ;
#78624=EDGE_LOOP ( 'NONE', ( #39973, #17573, #44579, #5598 ) ) ;
#78632=CARTESIAN_POINT ( 'NONE',  ( -7.669759969481850348, 72.54466164532334460, 118.1076662423914883 ) ) ;
#78660=ORIENTED_EDGE ( 'NONE', *, *, #35756, .F. ) ;
#78672=VERTEX_POINT ( 'NONE', #81962 ) ;
#78687=CARTESIAN_POINT ( 'NONE',  ( 7.674859615925401002, 72.54855685995774195, 118.1073353992515393 ) ) ;
#78703=EDGE_LOOP ( 'NONE', ( #16645, #13335, #39651, #25406 ) ) ;
#78713=DIRECTION ( 'NONE',  ( 0.000000000000000000, -1.000000000000000000, 0.000000000000000000 ) ) ;
#78737=PLANE ( 'NONE',  #71899 ) ;
#78771=DIRECTION ( 'NONE',  ( -0.9419738712670564507, -0.000000000000000000, -0.3356862014592719157 ) ) ;
#78775=DIRECTION ( 'NONE',  ( 0.000000000000000000, 0.000000000000000000, 1.000000000000000000 ) ) ;
#78821=ORIENTED_EDGE ( 'NONE', *, *, #84282, .T. ) ;
#78891=EDGE_CURVE ( 'NONE', #6718, #85945, #33912, .T. ) ;
#78895=EDGE_LOOP ( 'NONE', ( #25902, #57422, #7052, #44792 ) ) ;
#78898=ORIENTED_EDGE ( 'NONE', *, *, #66482, .F. ) ;
#78920=CARTESIAN_POINT ( 'NONE',  ( -446.0240000000000009, 3.174999999999999822, 101.5999999999999943 ) ) ;
#78940=DIRECTION ( 'NONE',  ( 1.000000000000000000, 0.000000000000000000, 0.000000000000000000 ) ) ;
#78941=EDGE_CURVE ( 'NONE', #27915, #79779, #64192, .T. ) ;
#78955=VECTOR ( 'NONE', #13983, 1000.000000000000000 ) ;
#78962=ORIENTED_EDGE ( 'NONE', *, *, #26812, .F. ) ;
#78992=ORIENTED_EDGE ( 'NONE', *, *, #27227, .F. ) ;
#78995=VERTEX_POINT ( 'NONE', #67757 ) ;
#79014=CIRCLE ( 'NONE', #3588, 12.70000000000000107 ) ;
#79036=DIRECTION ( 'NONE',  ( 1.000000000000000000, 0.000000000000000000, 0.000000000000000000 ) ) ;
#79071=CARTESIAN_POINT ( 'NONE',  ( -240.5296158183964792, 14.28749999999982201, 95.25000000000000000 ) ) ;
#79089=CARTESIAN_POINT ( 'NONE',  ( -492.0614999999999668, 93.66249999999999432, 15.87500000000039968 ) ) ;
#79096=VECTOR ( 'NONE', #35594, 1000.000000000000000 ) ;
#79110=CARTESIAN_POINT ( 'NONE',  ( 6.162975822039154730E-30, 95.25000000000000000, 118.5560000000000116 ) ) ;
#79118=ORIENTED_EDGE ( 'NONE', *, *, #82516, .T. ) ;
#79147=AXIS2_PLACEMENT_3D ( 'NONE', #64046, #84951, #37679 ) ;
#79177=DIRECTION ( 'NONE',  ( -0.000000000000000000, 0.8660254037844340447, 0.5000000000000081046 ) ) ;
#79178=EDGE_CURVE ( 'NONE', #30549, #31278, #46524, .T. ) ;
#79184=EDGE_CURVE ( 'NONE', #29469, #80801, #3558, .T. ) ;
#79185=CARTESIAN_POINT ( 'NONE',  ( -240.5296158183964792, 14.28749999999982201, 90.48749999999999716 ) ) ;
#79191=ORIENTED_EDGE ( 'NONE', *, *, #45548, .T. ) ;
#79215=DIRECTION ( 'NONE',  ( 0.000000000000000000, -1.000000000000000000, 0.000000000000000000 ) ) ;
#79226=CARTESIAN_POINT ( 'NONE',  ( -492.0614999999999668, 14.28750000000029985, 6.349999999999710099 ) ) ;
#79234=DIRECTION ( 'NONE',  ( 0.000000000000000000, 0.000000000000000000, -1.000000000000000000 ) ) ;
#79251=FACE_OUTER_BOUND ( 'NONE', #13263, .T. ) ;
#79286=DIRECTION ( 'NONE',  ( -0.8473160576754937834, 0.4185024680272297348, 0.3269727552264514725 ) ) ;
#79323=DIRECTION ( 'NONE',  ( 0.9130365726098601531, 0.000000000000000000, 0.4078776986755215384 ) ) ;
#79343=VERTEX_POINT ( 'NONE', #72692 ) ;
#79361=B_SPLINE_CURVE_WITH_KNOTS ( 'NONE', 1,
 ( #20692, #42453 ),
 .UNSPECIFIED., .F., .F.,
 ( 2, 2 ),
 ( 0.000000000000000000, 0.003789203591536580672 ),
 .UNSPECIFIED. ) ;
#79394=EDGE_LOOP ( 'NONE', ( #12591, #60461, #80390, #79191, #67146, #55952 ) ) ;
#79409=EDGE_LOOP ( 'NONE', ( #60889, #39196, #40620, #31150 ) ) ;
#79420=LINE ( 'NONE', #23562, #83485 ) ;
#79429=CARTESIAN_POINT ( 'NONE',  ( -41.60202597009397607, 40.59999999999997300, 50.85338361873603219 ) ) ;
#79434=ORIENTED_EDGE ( 'NONE', *, *, #59617, .F. ) ;
#79457=ADVANCED_FACE ( 'NONE', ( #65851 ), #31338, .T. ) ;
#79460=CARTESIAN_POINT ( 'NONE',  ( 61.00843881761244347, 49.07499999999999574, -33.74458626278666884 ) ) ;
#79462=CARTESIAN_POINT ( 'NONE',  ( 0.000000000000000000, 82.54999999999999716, 92.46299999999996544 ) ) ;
#79505=DIRECTION ( 'NONE',  ( 7.570719237730591757E-15, 1.000000000000000000, 0.000000000000000000 ) ) ;
#79507=VECTOR ( 'NONE', #83244, 1000.000000000000000 ) ;
#79508=EDGE_CURVE ( 'NONE', #77207, #14208, #7118, .T. ) ;
#79530=PLANE ( 'NONE',  #37505 ) ;
#79589=LINE ( 'NONE', #80933, #9631 ) ;
#79652=EDGE_CURVE ( 'NONE', #52534, #7158, #65986, .T. ) ;
#79659=CARTESIAN_POINT ( 'NONE',  ( -46.60773131249376888, 65.60000000000000853, -44.42500552774628630 ) ) ;
#79733=ORIENTED_EDGE ( 'NONE', *, *, #46536, .T. ) ;
#79743=FACE_OUTER_BOUND ( 'NONE', #531, .T. ) ;
#79746=EDGE_LOOP ( 'NONE', ( #8482, #45618, #51727, #14441 ) ) ;
#79761=ORIENTED_EDGE ( 'NONE', *, *, #69808, .F. ) ;
#79764=VERTEX_POINT ( 'NONE', #4762 ) ;
#79766=DIRECTION ( 'NONE',  ( 0.000000000000000000, 1.000000000000000000, 0.000000000000000000 ) ) ;
#79769=DIRECTION ( 'NONE',  ( 0.000000000000000000, 0.000000000000000000, 1.000000000000000000 ) ) ;
#79779=VERTEX_POINT ( 'NONE', #6114 ) ;
#79788=LINE ( 'NONE', #53363, #41627 ) ;
#79805=ORIENTED_EDGE ( 'NONE', *, *, #18652, .F. ) ;
#79816=DIRECTION ( 'NONE',  ( 0.000000000000000000, 0.000000000000000000, -1.000000000000000000 ) ) ;
#79821=CIRCLE ( 'NONE', #37736, 118.5560000000000116 ) ;
#79822=EDGE_LOOP ( 'NONE', ( #51599, #48908, #1834, #85365, #89921, #23946, #26261, #5836 ) ) ;
#79835=CARTESIAN_POINT ( 'NONE',  ( -487.2989999999999782, 93.66249999999999432, 95.25000000000000000 ) ) ;
#79837=LINE ( 'NONE', #10760, #1952 ) ;
#79859=CIRCLE ( 'NONE', #40661, 12.70000000000000107 ) ;
#79875=DIRECTION ( 'NONE',  ( -0.000000000000000000, -1.000000000000000000, -0.000000000000000000 ) ) ;
#79877=CARTESIAN_POINT ( 'NONE',  ( -479.3614999999999782, 93.66249999999999432, 98.73639197104678544 ) ) ;
#79887=EDGE_LOOP ( 'NONE', ( #38087, #87597, #86831, #50825 ) ) ;
#79891=DIRECTION ( 'NONE',  ( 1.000000000000000000, 0.000000000000000000, 0.000000000000000000 ) ) ;
#79912=LINE ( 'NONE', #57649, #69070 ) ;
#79916=EDGE_LOOP ( 'NONE', ( #7790, #34644, #74135, #89385 ) ) ;
#79919=ORIENTED_EDGE ( 'NONE', *, *, #12576, .F. ) ;
#79938=LINE ( 'NONE', #73541, #67912 ) ;
#79969=DIRECTION ( 'NONE',  ( 0.000000000000000000, 0.000000000000000000, 1.000000000000000000 ) ) ;
#79984=ORIENTED_EDGE ( 'NONE', *, *, #79652, .F. ) ;
#80005=CARTESIAN_POINT ( 'NONE',  ( 10.78439996481962915, 89.27017318066090468, 118.0647117534048647 ) ) ;
#80021=ORIENTED_EDGE ( 'NONE', *, *, #771, .T. ) ;
#80023=DIRECTION ( 'NONE',  ( 0.000000000000000000, -1.000000000000000000, 0.000000000000000000 ) ) ;
#80033=EDGE_CURVE ( 'NONE', #28457, #76903, #71431, .T. ) ;
#80077=EDGE_LOOP ( 'NONE', ( #67354, #10282, #34068 ) ) ;
#80095=ORIENTED_EDGE ( 'NONE', *, *, #83539, .F. ) ;
#80107=CARTESIAN_POINT ( 'NONE',  ( -6.360108159902766012, 71.54942407907350344, 118.3858500351901029 ) ) ;
#80128=DIRECTION ( 'NONE',  ( -1.776356839400250465E-15, 0.000000000000000000, -1.000000000000000000 ) ) ;
#80140=ORIENTED_EDGE ( 'NONE', *, *, #58795, .F. ) ;
#80141=ORIENTED_EDGE ( 'NONE', *, *, #39206, .F. ) ;
#80165=DIRECTION ( 'NONE',  ( -0.000000000000000000, 1.000000000000000000, -0.000000000000000000 ) ) ;
#80175=DIRECTION ( 'NONE',  ( 1.000000000000000000, 0.000000000000000000, 0.000000000000000000 ) ) ;
#80177=VERTEX_POINT ( 'NONE', #66593 ) ;
#80187=FACE_BOUND ( 'NONE', #18099, .T. ) ;
#80265=ORIENTED_EDGE ( 'NONE', *, *, #51455, .T. ) ;
#80312=EDGE_LOOP ( 'NONE', ( #66448, #29272, #4958, #19943 ) ) ;
#80317=DIRECTION ( 'NONE',  ( 0.000000000000000000, 0.8660254037844383745, -0.5000000000000003331 ) ) ;
#80390=ORIENTED_EDGE ( 'NONE', *, *, #42084, .T. ) ;
#80402=VERTEX_POINT ( 'NONE', #38672 ) ;
#80431=( GEOMETRIC_REPRESENTATION_CONTEXT ( 3 ) GLOBAL_UNCERTAINTY_ASSIGNED_CONTEXT ( ( #29649 ) ) GLOBAL_UNIT_ASSIGNED_CONTEXT ( ( #8131, #21772, #85796 ) ) REPRESENTATION_CONTEXT ( 'NONE', 'WORKASPACE' ) );
#80442=CARTESIAN_POINT ( 'NONE',  ( 12.37156061772173388, 85.44992509219818544, 117.9087631476423041 ) ) ;
#80498=VECTOR ( 'NONE', #88180, 1000.000000000000000 ) ;
#80523=FACE_BOUND ( 'NONE', #61708, .T. ) ;
#80545=DIRECTION ( 'NONE',  ( 0.000000000000000000, 0.000000000000000000, -1.000000000000000000 ) ) ;
#80550=EDGE_LOOP ( 'NONE', ( #70275, #6754, #2259, #82199 ) ) ;
#80568=ADVANCED_FACE ( 'NONE', ( #50865 ), #78154, .T. ) ;
#80570=DIRECTION ( 'NONE',  ( 0.2011513310014971800, -0.7071067811865459074, 0.6778924265960850626 ) ) ;
#80571=ADVANCED_FACE ( 'NONE', ( #15014, #3175 ), #22281, .T. ) ;
#80666=DIRECTION ( 'NONE',  ( 0.9586846635221889512, 0.000000000000000000, -0.2844709403917162205 ) ) ;
#80667=DIRECTION ( 'NONE',  ( -1.000000000000000000, 0.000000000000000000, 0.000000000000000000 ) ) ;
#80703=ORIENTED_EDGE ( 'NONE', *, *, #71559, .F. ) ;
#80728=DIRECTION ( 'NONE',  ( 0.000000000000000000, -0.4999999999999990563, -0.8660254037844392627 ) ) ;
#80731=FACE_OUTER_BOUND ( 'NONE', #19077, .T. ) ;
#80735=ORIENTED_EDGE ( 'NONE', *, *, #75535, .F. ) ;
#80779=DIRECTION ( 'NONE',  ( 1.000000000000000000, 0.000000000000000000, 0.000000000000000000 ) ) ;
#80781=CARTESIAN_POINT ( 'NONE',  ( -487.2989999999999782, 97.78694598552380057, 3.968750000000479616 ) ) ;
#80801=VERTEX_POINT ( 'NONE', #18572 ) ;
#80832=ORIENTED_EDGE ( 'NONE', *, *, #44877, .F. ) ;
#80846=CIRCLE ( 'NONE', #85197, 10.00000000000000178 ) ;
#80879=EDGE_CURVE ( 'NONE', #1571, #11233, #19940, .T. ) ;
#80885=AXIS2_PLACEMENT_3D ( 'NONE', #75021, #33689, #12352 ) ;
#80894=DIRECTION ( 'NONE',  ( 0.000000000000000000, 0.000000000000000000, -1.000000000000000000 ) ) ;
#80911=LINE ( 'NONE', #74518, #20964 ) ;
#80933=CARTESIAN_POINT ( 'NONE',  ( -487.2989999999999782, 18.41194598552320016, 97.63125000000000853 ) ) ;
#80944=ORIENTED_EDGE ( 'NONE', *, *, #20206, .T. ) ;
#80981=CIRCLE ( 'NONE', #2656, 16.33514202138213633 ) ;
#81001=CARTESIAN_POINT ( 'NONE',  ( -46.60773131249376178, 65.60000000000000853, -44.42500552774628630 ) ) ;
#81006=DIRECTION ( 'NONE',  ( 1.000000000000000000, 0.000000000000000000, 0.000000000000000000 ) ) ;
#81039=CARTESIAN_POINT ( 'NONE',  ( -492.0614999999999668, 93.66249999999999432, 6.350000000000409983 ) ) ;
#81042=DIRECTION ( 'NONE',  ( 0.000000000000000000, -0.000000000000000000, -1.000000000000000000 ) ) ;
#81063=( LENGTH_UNIT ( ) NAMED_UNIT ( * ) SI_UNIT ( .MILLI., .METRE. ) );
#81073=CARTESIAN_POINT ( 'NONE',  ( -492.0614999999999668, 14.28750000000026077, 11.11249999999970051 ) ) ;
#81076=AXIS2_PLACEMENT_3D ( 'NONE', #42368, #34671, #7870 ) ;
#81115=LINE ( 'NONE', #46983, #17513 ) ;
#81117=EDGE_CURVE ( 'NONE', #24603, #4807, #63447, .T. ) ;
#81138=AXIS2_PLACEMENT_3D ( 'NONE', #6868, #27760, #41815 ) ;
#81204=CARTESIAN_POINT ( 'NONE',  ( -24.20305689751608824, 54.97499999999995879, 58.62596543806478877 ) ) ;
#81228=CARTESIAN_POINT ( 'NONE',  ( -487.2989999999999782, 14.28750000000026077, 11.11249999999970051 ) ) ;
#81237=CARTESIAN_POINT ( 'NONE',  ( -7.399411900505344697, 92.88009567113228115, 118.3253705404784739 ) ) ;
#81257=VERTEX_POINT ( 'NONE', #30764 ) ;
#81272=AXIS2_PLACEMENT_3D ( 'NONE', #87074, #38452, #24840 ) ;
#81290=DIRECTION ( 'NONE',  ( 0.8660254037844432595, 0.4999999999999921174, 0.000000000000000000 ) ) ;
#81313=ORIENTED_EDGE ( 'NONE', *, *, #58084, .F. ) ;
#81328=AXIS2_PLACEMENT_3D ( 'NONE', #16986, #51476, #85598 ) ;
#81341=ORIENTED_EDGE ( 'NONE', *, *, #81117, .T. ) ;
#81370=CIRCLE ( 'NONE', #61037, 87.89999999999997726 ) ;
#81457=DIRECTION ( 'NONE',  ( 1.000000000000000000, 0.000000000000000000, 0.000000000000000000 ) ) ;
#81470=CARTESIAN_POINT ( 'NONE',  ( -10.00075923923900589, 90.22574527804057709, 117.9330208250991490 ) ) ;
#81473=ORIENTED_EDGE ( 'NONE', *, *, #79184, .T. ) ;
#81478=AXIS2_PLACEMENT_3D ( 'NONE', #40252, #54755, #33889 ) ;
#81502=ORIENTED_EDGE ( 'NONE', *, *, #71171, .F. ) ;
#81507=CIRCLE ( 'NONE', #56830, 38.10000000000000142 ) ;
#81536=FACE_OUTER_BOUND ( 'NONE', #89904, .T. ) ;
#81539=AXIS2_PLACEMENT_3D ( 'NONE', #37215, #66236, #2704 ) ;
#81556=ORIENTED_EDGE ( 'NONE', *, *, #1949, .F. ) ;
#81563=CARTESIAN_POINT ( 'NONE',  ( 0.000000000000000000, 93.07500000000001705, 88.90000000000000568 ) ) ;
#81575=DIRECTION ( 'NONE',  ( 0.000000000000000000, 0.8660254037844390407, -0.4999999999999995004 ) ) ;
#81611=LINE ( 'NONE', #59776, #43820 ) ;
#81618=CARTESIAN_POINT ( 'NONE',  ( -446.0240000000000009, 53.97500000000000142, 50.79999999999999716 ) ) ;
#81658=ORIENTED_EDGE ( 'NONE', *, *, #23094, .F. ) ;
#81661=CARTESIAN_POINT ( 'NONE',  ( 0.000000000000000000, 65.60000000000000853, 0.000000000000000000 ) ) ;
#81696=CARTESIAN_POINT ( 'NONE',  ( -41.60202597009397607, 65.59999999999998010, 47.15338361873602935 ) ) ;
#81729=VERTEX_POINT ( 'NONE', #12445 ) ;
#81759=CIRCLE ( 'NONE', #25195, 88.90000000000000568 ) ;
#81778=LINE ( 'NONE', #11380, #62429 ) ;
#81783=DIRECTION ( 'NONE',  ( 0.000000000000000000, 0.000000000000000000, -1.000000000000000000 ) ) ;
#81838=LINE ( 'NONE', #61808, #38860 ) ;
#81910=CARTESIAN_POINT ( 'NONE',  ( -5.572224674611368833, 93.85841628716941898, 118.2253171978965867 ) ) ;
#81918=DIRECTION ( 'NONE',  ( 0.9130365726098601531, 0.000000000000000000, 0.4078776986755215384 ) ) ;
#81939=VECTOR ( 'NONE', #29142, 1000.000000000000000 ) ;
#81954=PRESENTATION_STYLE_ASSIGNMENT (( #54192 ) ) ;
#81962=CARTESIAN_POINT ( 'NONE',  ( -487.2989999999999782, 89.53805401447711176, 3.968750000000410338 ) ) ;
#81996=VECTOR ( 'NONE', #77616, 1000.000000000000000 ) ;
#82007=EDGE_CURVE ( 'NONE', #57667, #1571, #60589, .T. ) ;
#82039=ORIENTED_EDGE ( 'NONE', *, *, #58795, .T. ) ;
#82063=CONICAL_SURFACE ( 'NONE', #31256, 118.5560000000000116, 0.7853981633974346233 ) ;
#82069=CARTESIAN_POINT ( 'NONE',  ( 0.000000000000000000, 82.54999999999999716, 92.46299999999996544 ) ) ;
#82071=DIRECTION ( 'NONE',  ( 0.000000000000000000, -5.300584669389750404E-15, 1.000000000000000000 ) ) ;
#82074=CYLINDRICAL_SURFACE ( 'NONE', #45313, 11.17600000000001970 ) ;
#82081=CARTESIAN_POINT ( 'NONE',  ( -479.3614999999999782, 3.174999999999999822, -1.387778780781445991E-14 ) ) ;
#82096=EDGE_CURVE ( 'NONE', #19571, #80402, #48289, .T. ) ;
#82101=CARTESIAN_POINT ( 'NONE',  ( -446.0240000000000009, 93.66249999999999432, 6.350000000000409983 ) ) ;
#82110=CARTESIAN_POINT ( 'NONE',  ( -47.11752803141010304, 65.60000000000000853, 108.7909173056707317 ) ) ;
#82121=LINE ( 'NONE', #768, #66135 ) ;
#82158=CARTESIAN_POINT ( 'NONE',  ( -487.2989999999999782, 86.51875000000001137, 86.36305401447658880 ) ) ;
#82164=CARTESIAN_POINT ( 'NONE',  ( 12.60000000000000142, 82.54999999999999716, 117.6834004267381744 ) ) ;
#82179=DIRECTION ( 'NONE',  ( 0.000000000000000000, 1.365923996832131856E-16, -1.000000000000000000 ) ) ;
#82181=FACE_OUTER_BOUND ( 'NONE', #84899, .T. ) ;
#82199=ORIENTED_EDGE ( 'NONE', *, *, #64682, .T. ) ;
#82205=CARTESIAN_POINT ( 'NONE',  ( -47.02966122971776741, 101.5999999999999943, 76.61736725193563302 ) ) ;
#82223=ADVANCED_FACE ( 'NONE', ( #10119 ), #78737, .F. ) ;
#82225=CARTESIAN_POINT ( 'NONE',  ( -74.84259178415759095, 53.97499999999998010, 30.79999999999997939 ) ) ;
#82226=EDGE_LOOP ( 'NONE', ( #43940, #82494, #88807, #16817 ) ) ;
#82275=ORIENTED_EDGE ( 'NONE', *, *, #70123, .F. ) ;
#82326=DIRECTION ( 'NONE',  ( 0.8861241255175470455, 0.000000000000000000, -0.4634479843259246556 ) ) ;
#82334=VECTOR ( 'NONE', #73255, 1000.000000000000000 ) ;
#82337=ORIENTED_EDGE ( 'NONE', *, *, #1209, .T. ) ;
#82360=CARTESIAN_POINT ( 'NONE',  ( -11.93750983681333899, 86.60304284441519940, 117.7525081508920408 ) ) ;
#82368=DIRECTION ( 'NONE',  ( 0.000000000000000000, 0.000000000000000000, -1.000000000000000000 ) ) ;
#82391=ORIENTED_EDGE ( 'NONE', *, *, #13796, .T. ) ;
#82413=EDGE_CURVE ( 'NONE', #77919, #36708, #32780, .T. ) ;
#82414=LINE ( 'NONE', #87869, #43397 ) ;
#82441=CARTESIAN_POINT ( 'NONE',  ( -47.02966122971774610, 92.07499999999998863, 74.26049396966043048 ) ) ;
#82460=DIRECTION ( 'NONE',  ( 0.000000000000000000, -0.4999999999999921174, -0.8660254037844431485 ) ) ;
#82467=DIRECTION ( 'NONE',  ( -1.000000000000000000, 0.000000000000000000, 0.000000000000000000 ) ) ;
#82494=ORIENTED_EDGE ( 'NONE', *, *, #83547, .T. ) ;
#82511=VECTOR ( 'NONE', #35064, 1000.000000000000000 ) ;
#82516=EDGE_CURVE ( 'NONE', #50313, #66470, #22622, .T. ) ;
#82525=EDGE_CURVE ( 'NONE', #12182, #65108, #21415, .T. ) ;
#82546=ADVANCED_FACE ( 'NONE', ( #70462 ), #41382, .F. ) ;
#82548=VERTEX_POINT ( 'NONE', #35023 ) ;
#82556=DIRECTION ( 'NONE',  ( 0.000000000000000000, 0.4999999999999897304, 0.8660254037844445918 ) ) ;
#82597=ORIENTED_EDGE ( 'NONE', *, *, #33681, .F. ) ;
#82609=DIRECTION ( 'NONE',  ( 0.000000000000000000, 0.000000000000000000, 1.000000000000000000 ) ) ;
#82616=PLANE ( 'NONE',  #60571 ) ;
#82631=PLANE ( 'NONE',  #32335 ) ;
#82648=EDGE_CURVE ( 'NONE', #55378, #83168, #36391, .T. ) ;
#82662=VERTEX_POINT ( 'NONE', #64981 ) ;
#82732=EDGE_CURVE ( 'NONE', #71111, #71979, #72247, .T. ) ;
#82744=EDGE_LOOP ( 'NONE', ( #9593, #40124, #36711, #19331 ) ) ;
#82748=AXIS2_PLACEMENT_3D ( 'NONE', #5471, #59065, #81783 ) ;
#82749=DIRECTION ( 'NONE',  ( 0.000000000000000000, 1.000000000000000000, 0.000000000000000000 ) ) ;
#82778=LINE ( 'NONE', #27336, #83825 ) ;
#82788=CARTESIAN_POINT ( 'NONE',  ( -492.0614999999999668, 14.28749999999982201, 85.72499999999999432 ) ) ;
#82806=LINE ( 'NONE', #63233, #82511 ) ;
#82821=CARTESIAN_POINT ( 'NONE',  ( -240.5296158183964792, 93.66249999999999432, 90.48749999999999716 ) ) ;
#82829=ORIENTED_EDGE ( 'NONE', *, *, #23034, .T. ) ;
#82833=VECTOR ( 'NONE', #38890, 1000.000000000000000 ) ;
#82859=VECTOR ( 'NONE', #39601, 1000.000000000000000 ) ;
#82863=DIRECTION ( 'NONE',  ( 0.6960018342484241005, 0.6960018342484289855, -0.1765301488291779741 ) ) ;
#82930=ORIENTED_EDGE ( 'NONE', *, *, #32572, .T. ) ;
#82946=ORIENTED_EDGE ( 'NONE', *, *, #28911, .F. ) ;
#83008=EDGE_CURVE ( 'NONE', #37391, #27515, #56040, .T. ) ;
#83019=VECTOR ( 'NONE', #360, 1000.000000000000000 ) ;
#83027=EDGE_CURVE ( 'NONE', #39332, #72160, #77960, .T. ) ;
#83066=CARTESIAN_POINT ( 'NONE',  ( 69.55653269757553403, 92.18234976669049274, 53.91899401579343731 ) ) ;
#83103=ORIENTED_EDGE ( 'NONE', *, *, #67059, .F. ) ;
#83133=EDGE_LOOP ( 'NONE', ( #38947, #19150, #29769, #60166 ) ) ;
#83168=VERTEX_POINT ( 'NONE', #85677 ) ;
#83205=CARTESIAN_POINT ( 'NONE',  ( -479.3614999999999782, 89.53805401447711176, 3.968750000000410338 ) ) ;
#83244=DIRECTION ( 'NONE',  ( 0.2884130866282269556, 0.7071067811865447972, -0.6456143519637576045 ) ) ;
#83265=ORIENTED_EDGE ( 'NONE', *, *, #82648, .T. ) ;
#83277=CARTESIAN_POINT ( 'NONE',  ( -479.3614999999999782, 97.78694598552380057, 3.968750000000479616 ) ) ;
#83290=DIRECTION ( 'NONE',  ( 1.000000000000000000, 0.000000000000000000, 0.000000000000000000 ) ) ;
#83297=DIRECTION ( 'NONE',  ( 0.000000000000000000, 0.000000000000000000, 1.000000000000000000 ) ) ;
#83309=EDGE_CURVE ( 'NONE', #52469, #67042, #5674, .T. ) ;
#83321=CARTESIAN_POINT ( 'NONE',  ( -41.60202597009397607, 65.59999999999998010, 54.55338361873603503 ) ) ;
#83334=EDGE_CURVE ( 'NONE', #7646, #65744, #6121, .T. ) ;
#83342=VERTEX_POINT ( 'NONE', #25652 ) ;
#83349=VECTOR ( 'NONE', #1211, 1000.000000000000000 ) ;
#83365=ORIENTED_EDGE ( 'NONE', *, *, #76003, .F. ) ;
#83396=DIRECTION ( 'NONE',  ( 0.000000000000000000, 0.000000000000000000, 1.000000000000000000 ) ) ;
#83403=FACE_OUTER_BOUND ( 'NONE', #80312, .T. ) ;
#83419=AXIS2_PLACEMENT_3D ( 'NONE', #39054, #88121, #4988 ) ;
#83447=ORIENTED_EDGE ( 'NONE', *, *, #83547, .F. ) ;
#83460=ORIENTED_EDGE ( 'NONE', *, *, #55169, .F. ) ;
#83485=VECTOR ( 'NONE', #70805, 1000.000000000000000 ) ;
#83493=DIRECTION ( 'NONE',  ( 1.000000000000000000, 0.000000000000000000, 0.000000000000000000 ) ) ;
#83496=CARTESIAN_POINT ( 'NONE',  ( 69.13171461148455421, 92.73732945906610325, 55.35424314442764882 ) ) ;
#83532=EDGE_CURVE ( 'NONE', #55523, #69100, #55119, .T. ) ;
#83539=EDGE_CURVE ( 'NONE', #1472, #56124, #20642, .T. ) ;
#83547=EDGE_CURVE ( 'NONE', #49587, #81729, #89689, .T. ) ;
#83591=VERTEX_POINT ( 'NONE', #65096 ) ;
#83593=EDGE_LOOP ( 'NONE', ( #50928, #12096, #63807 ) ) ;
#83599=CARTESIAN_POINT ( 'NONE',  ( -254.0000000000000000, 14.28750000000026077, 11.11249999999970051 ) ) ;
#83627=CARTESIAN_POINT ( 'NONE',  ( 0.000000000000000000, 65.60000000000000853, 118.5560000000000116 ) ) ;
#83639=ADVANCED_FACE ( 'NONE', ( #36942 ), #68403, .T. ) ;
#83653=CARTESIAN_POINT ( 'NONE',  ( -47.02966122971771767, 65.60000000000000853, -44.00307561052230199 ) ) ;
#83663=EDGE_CURVE ( 'NONE', #19584, #37970, #60957, .T. ) ;
#83680=DIRECTION ( 'NONE',  ( 0.000000000000000000, 0.000000000000000000, -1.000000000000000000 ) ) ;
#83682=CARTESIAN_POINT ( 'NONE',  ( 2.061567565891823328, 94.98702740777858367, 118.3387339768891593 ) ) ;
#83685=EDGE_CURVE ( 'NONE', #77202, #21144, #25996, .T. ) ;
#83690=ADVANCED_FACE ( 'NONE', ( #59594 ), #87331, .F. ) ;
#83694=ORIENTED_EDGE ( 'NONE', *, *, #8054, .F. ) ;
#83697=ORIENTED_EDGE ( 'NONE', *, *, #7956, .F. ) ;
#83708=EDGE_CURVE ( 'NONE', #7908, #87146, #12366, .T. ) ;
#83790=CARTESIAN_POINT ( 'NONE',  ( -479.3614999999999782, 100.8062500000000057, 86.36305401447658880 ) ) ;
#83820=AXIS2_PLACEMENT_3D ( 'NONE', #3942, #66608, #4399 ) ;
#83825=VECTOR ( 'NONE', #29140, 1000.000000000000000 ) ;
#83829=VERTEX_POINT ( 'NONE', #69570 ) ;
#83845=ORIENTED_EDGE ( 'NONE', *, *, #4282, .F. ) ;
#83855=CARTESIAN_POINT ( 'NONE',  ( -487.2989999999999782, 10.16305401447644030, 97.63125000000000853 ) ) ;
#83892=VECTOR ( 'NONE', #44887, 1000.000000000000114 ) ;
#83906=LINE ( 'NONE', #23471, #39884 ) ;
#83961=LINE ( 'NONE', #49404, #32041 ) ;
#84006=CARTESIAN_POINT ( 'NONE',  ( -76.66819259232177330, 55.29345935402049150, 30.84311214076278773 ) ) ;
#84017=VECTOR ( 'NONE', #76789, 1000.000000000000000 ) ;
#84028=CARTESIAN_POINT ( 'NONE',  ( -215.9000000000000057, 3.174999999999999822, -41.27499999999999858 ) ) ;
#84041=ORIENTED_EDGE ( 'NONE', *, *, #31797, .F. ) ;
#84046=DIRECTION ( 'NONE',  ( 1.000000000000000000, 0.000000000000000000, 0.000000000000000000 ) ) ;
#84055=CARTESIAN_POINT ( 'NONE',  ( 1.796236281188243881E-22, 69.84999999999999432, 118.5560000000000116 ) ) ;
#84062=CIRCLE ( 'NONE', #40465, 4.762500000000002842 ) ;
#84093=EDGE_LOOP ( 'NONE', ( #34163, #78332, #1242, #214, #63879, #12523, #21583 ) ) ;
#84099=DIRECTION ( 'NONE',  ( 0.000000000000000000, 1.000000000000000000, 1.047445008332813989E-14 ) ) ;
#84107=LINE ( 'NONE', #83653, #49073 ) ;
#84131=AXIS2_PLACEMENT_3D ( 'NONE', #82821, #34188, #34643 ) ;
#84138=ORIENTED_EDGE ( 'NONE', *, *, #63009, .F. ) ;
#84196=DIRECTION ( 'NONE',  ( 0.000000000000000000, -1.000000000000000000, 0.000000000000000000 ) ) ;
#84225=ORIENTED_EDGE ( 'NONE', *, *, #18652, .T. ) ;
#84270=DIRECTION ( 'NONE',  ( 1.000000000000000000, 0.000000000000000000, 0.000000000000000000 ) ) ;
#84282=EDGE_CURVE ( 'NONE', #29846, #59106, #40406, .T. ) ;
#84353=EDGE_CURVE ( 'NONE', #71979, #2341, #61740, .T. ) ;
#84397=DIRECTION ( 'NONE',  ( 0.000000000000000000, 0.7071067811865671127, 0.7071067811865279218 ) ) ;
#84439=VERTEX_POINT ( 'NONE', #56251 ) ;
#84441=ORIENTED_EDGE ( 'NONE', *, *, #34464, .F. ) ;
#84499=VECTOR ( 'NONE', #19778, 1000.000000000000000 ) ;
#84510=DIRECTION ( 'NONE',  ( 0.000000000000000000, 0.000000000000000000, 1.000000000000000000 ) ) ;
#84520=ORIENTED_EDGE ( 'NONE', *, *, #4086, .F. ) ;
#84579=DIRECTION ( 'NONE',  ( 1.000000000000000000, 0.000000000000000000, 0.000000000000000000 ) ) ;
#84588=CARTESIAN_POINT ( 'NONE',  ( 10.91422574807192625, 88.85956302702116716, 117.8518595483441800 ) ) ;
#84591=ORIENTED_EDGE ( 'NONE', *, *, #58355, .T. ) ;
#84653=CARTESIAN_POINT ( 'NONE',  ( -47.02966122971772478, 65.60000000000000853, -8.565507749926083175E-15 ) ) ;
#84671=DIRECTION ( 'NONE',  ( -1.000000000000000000, 0.000000000000000000, 0.000000000000000000 ) ) ;
#84707=AXIS2_PLACEMENT_3D ( 'NONE', #57355, #24194, #51425 ) ;
#84712=ORIENTED_EDGE ( 'NONE', *, *, #82525, .F. ) ;
#84714=EDGE_LOOP ( 'NONE', ( #37510, #5213, #15767, #756, #38176 ) ) ;
#84730=EDGE_LOOP ( 'NONE', ( #29304, #13927, #70365, #35432, #15672 ) ) ;
#84746=ORIENTED_EDGE ( 'NONE', *, *, #19132, .T. ) ;
#84753=DIRECTION ( 'NONE',  ( 1.000000000000000000, 0.000000000000000000, 0.000000000000000000 ) ) ;
#84759=LINE ( 'NONE', #77935, #571 ) ;
#84762=FACE_OUTER_BOUND ( 'NONE', #61355, .T. ) ;
#84771=CARTESIAN_POINT ( 'NONE',  ( -458.3598257906459708, 60.32499999999999574, 3.174999999999999822 ) ) ;
#84809=EDGE_CURVE ( 'NONE', #67327, #76187, #6683, .T. ) ;
#84831=EDGE_LOOP ( 'NONE', ( #48928, #7922, #1787, #47514, #14231 ) ) ;
#84840=VERTEX_POINT ( 'NONE', #11086 ) ;
#84841=CARTESIAN_POINT ( 'NONE',  ( 61.00843881761244347, 65.60000000000000853, -53.97512327982435210 ) ) ;
#84848=VECTOR ( 'NONE', #19550, 1000.000000000000000 ) ;
#84851=CONICAL_SURFACE ( 'NONE', #3587, 88.90000000000000568, 0.7853981633974552734 ) ;
#84869=VERTEX_POINT ( 'NONE', #73767 ) ;
#84878=DIRECTION ( 'NONE',  ( -1.000000000000000000, 0.000000000000000000, 0.000000000000000000 ) ) ;
#84894=CARTESIAN_POINT ( 'NONE',  ( -47.11752803141011015, 100.5999999999999659, 108.7909173056707317 ) ) ;
#84899=EDGE_LOOP ( 'NONE', ( #27453, #50248, #35351, #49069 ) ) ;
#84902=AXIS2_PLACEMENT_3D ( 'NONE', #78397, #2076, #1180 ) ;
#84905=ADVANCED_FACE ( 'NONE', ( #32411 ), #71958, .T. ) ;
#84908=CARTESIAN_POINT ( 'NONE',  ( -74.56320856954198462, 53.97500000000000142, 30.79999999999999361 ) ) ;
#84937=CARTESIAN_POINT ( 'NONE',  ( -55.89999999999999858, 53.97500000000000142, 70.79999999999999716 ) ) ;
#84951=DIRECTION ( 'NONE',  ( -0.000000000000000000, 1.000000000000000000, -0.000000000000000000 ) ) ;
#84957=CARTESIAN_POINT ( 'NONE',  ( 12.27439874544222853, 79.26318322085235479, 117.9189513481508982 ) ) ;
#85039=CARTESIAN_POINT ( 'NONE',  ( -34.93928583487483763, 53.97499999999997300, 35.93880153443800651 ) ) ;
#85045=CARTESIAN_POINT ( 'NONE',  ( 11.30815728993320413, 76.97724414224275336, 117.8147121273327684 ) ) ;
#85052=ADVANCED_FACE ( 'NONE', ( #51501, #79251 ), #51069, .T. ) ;
#85070=LINE ( 'NONE', #23733, #45428 ) ;
#85078=ORIENTED_EDGE ( 'NONE', *, *, #88559, .T. ) ;
#85093=LINE ( 'NONE', #45054, #23908 ) ;
#85100=CARTESIAN_POINT ( 'NONE',  ( -41.60202597009397607, 64.60000000000000853, 33.51824159735392783 ) ) ;
#85112=CIRCLE ( 'NONE', #16884, 39.10000000000005116 ) ;
#85119=ADVANCED_FACE ( 'NONE', ( #46471 ), #12423, .F. ) ;
#85139=DIRECTION ( 'NONE',  ( 0.000000000000000000, 0.000000000000000000, -1.000000000000000000 ) ) ;
#85143=CARTESIAN_POINT ( 'NONE',  ( -41.60202597009397607, 65.59999999999998010, 50.85338361873603219 ) ) ;
#85147=EDGE_LOOP ( 'NONE', ( #2678, #5561, #28181, #45562, #43339, #23220 ) ) ;
#85153=CONICAL_SURFACE ( 'NONE', #37280, 16.33514202138210791, 0.7853981633974552734 ) ;
#85179=AXIS2_PLACEMENT_3D ( 'NONE', #35286, #21689, #55268 ) ;
#85197=AXIS2_PLACEMENT_3D ( 'NONE', #56774, #71326, #85419 ) ;
#85201=EDGE_LOOP ( 'NONE', ( #67013, #30174, #27853, #87177, #48103 ) ) ;
#85234=EDGE_CURVE ( 'NONE', #14474, #27515, #12169, .T. ) ;
#85251=VECTOR ( 'NONE', #26690, 1000.000000000000000 ) ;
#85263=AXIS2_PLACEMENT_3D ( 'NONE', #14461, #19472, #83493 ) ;
#85333=LINE ( 'NONE', #30784, #32920 ) ;
#85338=ORIENTED_EDGE ( 'NONE', *, *, #30857, .F. ) ;
#85364=CARTESIAN_POINT ( 'NONE',  ( -479.3614999999999782, 89.53805401447711176, 3.968750000000410338 ) ) ;
#85365=ORIENTED_EDGE ( 'NONE', *, *, #35440, .T. ) ;
#85388=CARTESIAN_POINT ( 'NONE',  ( 61.00843881761244347, 65.60000000000000853, 0.000000000000000000 ) ) ;
#85419=DIRECTION ( 'NONE',  ( 0.000000000000000000, 0.000000000000000000, -1.000000000000000000 ) ) ;
#85440=CYLINDRICAL_SURFACE ( 'NONE', #76, 4.762500000000000178 ) ;
#85441=FACE_OUTER_BOUND ( 'NONE', #18802, .T. ) ;
#85459=CYLINDRICAL_SURFACE ( 'NONE', #27721, 3.814291549405317117 ) ;
#85485=DIRECTION ( 'NONE',  ( -0.000000000000000000, 1.000000000000000000, -0.000000000000000000 ) ) ;
#85498=AXIS2_PLACEMENT_3D ( 'NONE', #5029, #31381, #33181 ) ;
#85537=ORIENTED_EDGE ( 'NONE', *, *, #45195, .T. ) ;
#85566=CARTESIAN_POINT ( 'NONE',  ( -48.02966122971776741, 93.07500000000001705, 75.53254848357481421 ) ) ;
#85585=PLANE ( 'NONE',  #51997 ) ;
#85586=CARTESIAN_POINT ( 'NONE',  ( 68.86456684384336313, 93.07500000000001705, 56.22171674193015889 ) ) ;
#85598=DIRECTION ( 'NONE',  ( 0.000000000000000000, 0.000000000000000000, 1.000000000000000000 ) ) ;
#85611=VERTEX_POINT ( 'NONE', #25951 ) ;
#85621=ORIENTED_EDGE ( 'NONE', *, *, #39208, .T. ) ;
#85627=EDGE_CURVE ( 'NONE', #74649, #19571, #79589, .T. ) ;
#85647=CARTESIAN_POINT ( 'NONE',  ( 70.63919639214310564, 100.5999999999999659, 56.85413200336923012 ) ) ;
#85656=DIRECTION ( 'NONE',  ( -0.4428439315555359745, -0.8965987130731539745, 0.000000000000000000 ) ) ;
#85677=CARTESIAN_POINT ( 'NONE',  ( -254.0000000000000000, 53.97500000000000142, 0.000000000000000000 ) ) ;
#85678=ORIENTED_EDGE ( 'NONE', *, *, #33164, .T. ) ;
#85689=ADVANCED_FACE ( 'NONE', ( #53164 ), #50339, .F. ) ;
#85693=CARTESIAN_POINT ( 'NONE',  ( 0.000000000000000000, 92.07499999999998863, 0.000000000000000000 ) ) ;
#85710=CYLINDRICAL_SURFACE ( 'NONE', #12607, 118.5560000000000116 ) ;
#85745=EDGE_CURVE ( 'NONE', #80801, #29469, #34389, .T. ) ;
#85748=PLANE ( 'NONE',  #9704 ) ;
#85796=( NAMED_UNIT ( * ) SI_UNIT ( $, .STERADIAN. ) SOLID_ANGLE_UNIT ( ) );
#85874=AXIS2_PLACEMENT_3D ( 'NONE', #45099, #27688, #61741 ) ;
#85877=FACE_OUTER_BOUND ( 'NONE', #12436, .T. ) ;
#85889=FACE_OUTER_BOUND ( 'NONE', #57249, .T. ) ;
#85914=AXIS2_PLACEMENT_3D ( 'NONE', #393, #28087, #47631 ) ;
#85922=EDGE_CURVE ( 'NONE', #51377, #79343, #80846, .T. ) ;
#85945=VERTEX_POINT ( 'NONE', #36795 ) ;
#85956=CARTESIAN_POINT ( 'NONE',  ( -487.2989999999999782, 89.53805401447691281, 18.25625000000039933 ) ) ;
#86005=CIRCLE ( 'NONE', #55478, 118.5560000000000116 ) ;
#86024=LINE ( 'NONE', #65558, #51554 ) ;
#86033=CARTESIAN_POINT ( 'NONE',  ( 0.000000000000000000, 93.07500000000001705, 0.000000000000000000 ) ) ;
#86037=ORIENTED_EDGE ( 'NONE', *, *, #37622, .F. ) ;
#86066=VECTOR ( 'NONE', #42446, 1000.000000000000000 ) ;
#86094=PLANE ( 'NONE',  #15860 ) ;
#86106=DIRECTION ( 'NONE',  ( 0.000000000000000000, -1.000000000000000000, 0.000000000000000000 ) ) ;
#86124=VERTEX_POINT ( 'NONE', #11765 ) ;
#86132=CYLINDRICAL_SURFACE ( 'NONE', #50954, 88.90000000000000568 ) ;
#86149=TOROIDAL_SURFACE ( 'NONE', #67256, 36.57600000000000051, 1.524000000000000021 ) ;
#86151=ORIENTED_EDGE ( 'NONE', *, *, #75938, .T. ) ;
#86153=DIRECTION ( 'NONE',  ( -1.000000000000000000, 0.000000000000000000, 0.000000000000000000 ) ) ;
#86162=EDGE_CURVE ( 'NONE', #43418, #84840, #45365, .T. ) ;
#86179=LINE ( 'NONE', #58450, #66347 ) ;
#86255=DIRECTION ( 'NONE',  ( -1.000000000000000000, 0.000000000000000000, 0.000000000000000000 ) ) ;
#86298=ORIENTED_EDGE ( 'NONE', *, *, #32960, .F. ) ;
#86299=ADVANCED_FACE ( 'NONE', ( #60338 ), #19020, .T. ) ;
#86327=LINE ( 'NONE', #72701, #51415 ) ;
#86339=ADVANCED_FACE ( 'NONE', ( #20377 ), #82616, .F. ) ;
#86375=CARTESIAN_POINT ( 'NONE',  ( -446.0240000000000009, 93.66249999999999432, 95.25000000000000000 ) ) ;
#86386=DIRECTION ( 'NONE',  ( 0.000000000000000000, -1.000000000000000000, 0.000000000000000000 ) ) ;
#86397=CIRCLE ( 'NONE', #58817, 11.17600000000001970 ) ;
#86416=AXIS2_PLACEMENT_3D ( 'NONE', #61730, #27677, #27223 ) ;
#86433=ADVANCED_FACE ( 'NONE', ( #64392, #70765 ), #7633, .T. ) ;
#86474=CARTESIAN_POINT ( 'NONE',  ( -11.00083755277435138, 76.19034529151561230, 118.0446767648407302 ) ) ;
#86503=CARTESIAN_POINT ( 'NONE',  ( 70.30576339899383242, 100.9334329931492675, 95.04579496287460927 ) ) ;
#86511=EDGE_CURVE ( 'NONE', #72546, #15662, #86179, .T. ) ;
#86531=DIRECTION ( 'NONE',  ( -1.000000000000000000, 0.000000000000000000, 0.000000000000000000 ) ) ;
#86533=LINE ( 'NONE', #85647, #21547 ) ;
#86534=DIRECTION ( 'NONE',  ( -0.000000000000000000, 1.000000000000000000, -0.000000000000000000 ) ) ;
#86569=ORIENTED_EDGE ( 'NONE', *, *, #17419, .T. ) ;
#86583=CARTESIAN_POINT ( 'NONE',  ( -15.88716625750469902, 65.60000000000000853, -53.54073290201169044 ) ) ;
#86600=AXIS2_PLACEMENT_3D ( 'NONE', #55861, #40907, #36 ) ;
#86634=DIRECTION ( 'NONE',  ( 0.000000000000000000, 0.000000000000000000, 1.000000000000000000 ) ) ;
#86678=ADVANCED_FACE ( 'NONE', ( #73424, #17578 ), #66154, .T. ) ;
#86690=ADVANCED_FACE ( 'NONE', ( #72102 ), #9875, .F. ) ;
#86747=ORIENTED_EDGE ( 'NONE', *, *, #76725, .T. ) ;
#86766=DIRECTION ( 'NONE',  ( 0.000000000000000000, 0.000000000000000000, 1.000000000000000000 ) ) ;
#86775=DIRECTION ( 'NONE',  ( 0.000000000000000000, 0.000000000000000000, 1.000000000000000000 ) ) ;
#86783=EDGE_LOOP ( 'NONE', ( #67772, #52595, #81313 ) ) ;
#86814=CYLINDRICAL_SURFACE ( 'NONE', #85498, 4.762500000000002842 ) ;
#86831=ORIENTED_EDGE ( 'NONE', *, *, #48741, .F. ) ;
#86853=CIRCLE ( 'NONE', #49146, 4.762500000000000178 ) ;
#86906=PLANE ( 'NONE',  #33318 ) ;
#86911=ADVANCED_FACE ( 'NONE', ( #42032, #41576 ), #76113, .T. ) ;
#86912=CARTESIAN_POINT ( 'NONE',  ( -5.244729318936814266, 70.97606371242190448, 118.4405590227164851 ) ) ;
#86924=CARTESIAN_POINT ( 'NONE',  ( -215.9000000000000057, 3.174999999999999822, -41.27499999999999858 ) ) ;
#86942=CARTESIAN_POINT ( 'NONE',  ( -479.3614999999999782, 101.9113919710471947, 11.11250000000054072 ) ) ;
#86946=ORIENTED_EDGE ( 'NONE', *, *, #6679, .T. ) ;
#86964=CIRCLE ( 'NONE', #47774, 4.762499999999999289 ) ;
#87008=CIRCLE ( 'NONE', #63802, 16.33514202138213633 ) ;
#87051=ORIENTED_EDGE ( 'NONE', *, *, #31363, .F. ) ;
#87068=ORIENTED_EDGE ( 'NONE', *, *, #66474, .F. ) ;
#87074=CARTESIAN_POINT ( 'NONE',  ( -254.0000000000000000, 53.97500000000000142, 50.79999999999999716 ) ) ;
#87118=CARTESIAN_POINT ( 'NONE',  ( 0.000000000000000000, 91.07499999999996021, 0.000000000000000000 ) ) ;
#87119=DIRECTION ( 'NONE',  ( 0.000000000000000000, 0.000000000000000000, 1.000000000000000000 ) ) ;
#87131=EDGE_CURVE ( 'NONE', #40908, #274, #81838, .T. ) ;
#87140=CARTESIAN_POINT ( 'NONE',  ( 6.162975822039154730E-30, 95.25000000000000000, 118.5560000000000116 ) ) ;
#87146=VERTEX_POINT ( 'NONE', #5981 ) ;
#87151=CARTESIAN_POINT ( 'NONE',  ( -446.0240000000000009, 3.174999999999999822, 101.5999999999999943 ) ) ;
#87157=AXIS2_PLACEMENT_3D ( 'NONE', #62161, #12688, #76246 ) ;
#87177=ORIENTED_EDGE ( 'NONE', *, *, #80033, .F. ) ;
#87195=VECTOR ( 'NONE', #19179, 1000.000000000000000 ) ;
#87213=VERTEX_POINT ( 'NONE', #48611 ) ;
#87226=ADVANCED_FACE ( 'NONE', ( #76351 ), #41805, .F. ) ;
#87233=ADVANCED_FACE ( 'NONE', ( #47279 ), #26412, .T. ) ;
#87256=EDGE_LOOP ( 'NONE', ( #15820, #79984, #7312, #7303 ) ) ;
#87276=DIRECTION ( 'NONE',  ( 0.000000000000000000, 0.000000000000000000, 1.000000000000000000 ) ) ;
#87291=AXIS2_PLACEMENT_3D ( 'NONE', #15812, #9435, #16259 ) ;
#87316=EDGE_CURVE ( 'NONE', #83591, #36325, #78170, .T. ) ;
#87331=PLANE ( 'NONE',  #44239 ) ;
#87345=ORIENTED_EDGE ( 'NONE', *, *, #32562, .T. ) ;
#87369=CARTESIAN_POINT ( 'NONE',  ( -6.299534494109307659, 93.46997398832955639, 118.1887946445226589 ) ) ;
#87391=DIRECTION ( 'NONE',  ( 0.000000000000000000, -1.000000000000000000, -3.491483361109380094E-15 ) ) ;
#87443=DIRECTION ( 'NONE',  ( 0.000000000000000000, -1.000000000000000000, 0.000000000000000000 ) ) ;
#87454=VERTEX_POINT ( 'NONE', #60358 ) ;
#87473=DIRECTION ( 'NONE',  ( 0.2844709403917162205, 0.000000000000000000, 0.9586846635221889512 ) ) ;
#87486=DIRECTION ( 'NONE',  ( -0.000000000000000000, 1.000000000000000000, -0.000000000000000000 ) ) ;
#87489=DIRECTION ( 'NONE',  ( 0.000000000000000000, 0.000000000000000000, -1.000000000000000000 ) ) ;
#87523=LINE ( 'NONE', #25284, #40394 ) ;
#87536=LINE ( 'NONE', #66631, #45182 ) ;
#87541=CYLINDRICAL_SURFACE ( 'NONE', #31206, 1.999999999999999112 ) ;
#87582=CARTESIAN_POINT ( 'NONE',  ( -2.883663860655375721, 94.92521392225150123, 118.5216208257077710 ) ) ;
#87586=ORIENTED_EDGE ( 'NONE', *, *, #1949, .T. ) ;
#87592=EDGE_CURVE ( 'NONE', #54435, #57667, #59211, .T. ) ;
#87597=ORIENTED_EDGE ( 'NONE', *, *, #78023, .F. ) ;
#87598=ADVANCED_FACE ( 'NONE', ( #27644 ), #51935, .F. ) ;
#87660=PLANE ( 'NONE',  #68631 ) ;
#87671=CARTESIAN_POINT ( 'NONE',  ( -479.3614999999999782, 3.174999999999999822, 101.5999999999999943 ) ) ;
#87672=CARTESIAN_POINT ( 'NONE',  ( -254.0000000000000000, 3.174999999999999822, 142.8750000000000000 ) ) ;
#87698=CARTESIAN_POINT ( 'NONE',  ( 61.00843881761244347, 49.07499999999999574, -53.97512327982435210 ) ) ;
#87700=PLANE ( 'NONE',  #8586 ) ;
#87719=ORIENTED_EDGE ( 'NONE', *, *, #30016, .F. ) ;
#87752=AXIS2_PLACEMENT_3D ( 'NONE', #27822, #77325, #1023 ) ;
#87768=LINE ( 'NONE', #88679, #87195 ) ;
#87796=LINE ( 'NONE', #72826, #82334 ) ;
#87869=CARTESIAN_POINT ( 'NONE',  ( -47.16614613999456651, 91.93851508972313979, -43.22209291737998882 ) ) ;
#87903=SHAPE_REPRESENTATION ( 'Rotary Table Drive Mechanism', ( #50656 ), #27649 ) ;
#87906=AXIS2_PLACEMENT_3D ( 'NONE', #42279, #13253, #40939 ) ;
#87927=FACE_OUTER_BOUND ( 'NONE', #46316, .T. ) ;
#87940=AXIS2_PLACEMENT_3D ( 'NONE', #20995, #63673, #1457 ) ;
#87958=PLANE ( 'NONE',  #10751 ) ;
#87961=VERTEX_POINT ( 'NONE', #73896 ) ;
#88003=CYLINDRICAL_SURFACE ( 'NONE', #74346, 4.762500000000002842 ) ;
#88022=ORIENTED_EDGE ( 'NONE', *, *, #6926, .F. ) ;
#88030=ADVANCED_FACE ( 'NONE', ( #46166, #67079, #13912, #41592, #26196, #18934 ), #40260, .F. ) ;
#88066=EDGE_CURVE ( 'NONE', #67042, #75662, #13026, .T. ) ;
#88118=FACE_OUTER_BOUND ( 'NONE', #85147, .T. ) ;
#88121=DIRECTION ( 'NONE',  ( -1.000000000000000000, 0.000000000000000000, 0.000000000000000000 ) ) ;
#88130=ORIENTED_EDGE ( 'NONE', *, *, #5270, .F. ) ;
#88180=DIRECTION ( 'NONE',  ( 0.000000000000000000, 0.000000000000000000, 1.000000000000000000 ) ) ;
#88215=VECTOR ( 'NONE', #31454, 1000.000000000000000 ) ;
#88231=AXIS2_PLACEMENT_3D ( 'NONE', #40862, #46321, #89481 ) ;
#88241=DIRECTION ( 'NONE',  ( -0.9130365726098600421, 0.000000000000000000, -0.4078776986755216494 ) ) ;
#88253=ORIENTED_EDGE ( 'NONE', *, *, #71445, .T. ) ;
#88258=DIRECTION ( 'NONE',  ( 0.000000000000000000, 1.000000000000000000, 0.000000000000000000 ) ) ;
#88309=CARTESIAN_POINT ( 'NONE',  ( -479.3614999999999782, 97.78694598552370110, 18.25625000000050235 ) ) ;
#88331=CARTESIAN_POINT ( 'NONE',  ( -450.8499999999999659, 53.97500000000000142, -3.174999999999999822 ) ) ;
#88346=ADVANCED_FACE ( 'NONE', ( #84762 ), #22527, .T. ) ;
#88350=VECTOR ( 'NONE', #71420, 1000.000000000000000 ) ;
#88352=VERTEX_POINT ( 'NONE', #45599 ) ;
#88373=CARTESIAN_POINT ( 'NONE',  ( -479.3614999999999782, 101.9113919710471947, 11.11250000000054072 ) ) ;
#88377=ORIENTED_EDGE ( 'NONE', *, *, #64149, .T. ) ;
#88378=ADVANCED_FACE ( 'NONE', ( #65191 ), #86094, .T. ) ;
#88397=VERTEX_POINT ( 'NONE', #31549 ) ;
#88419=DIRECTION ( 'NONE',  ( 0.000000000000000000, 1.000000000000000000, 1.809101308280369915E-15 ) ) ;
#88424=DIRECTION ( 'NONE',  ( 0.000000000000000000, 1.000000000000000000, 0.000000000000000000 ) ) ;
#88434=LINE ( 'NONE', #10762, #19792 ) ;
#88472=DIRECTION ( 'NONE',  ( 0.000000000000000000, 0.000000000000000000, -1.000000000000000000 ) ) ;
#88488=CARTESIAN_POINT ( 'NONE',  ( -6.364298811279507362, 93.57154221663603266, 118.3870716450922629 ) ) ;
#88495=ORIENTED_EDGE ( 'NONE', *, *, #44070, .F. ) ;
#88559=EDGE_CURVE ( 'NONE', #52469, #77842, #82414, .T. ) ;
#88563=CARTESIAN_POINT ( 'NONE',  ( -47.08158946516970644, 101.2663385054221408, 76.19398627647811395 ) ) ;
#88565=ADVANCED_FACE ( 'NONE', ( #68769 ), #53308, .T. ) ;
#88593=CIRCLE ( 'NONE', #56616, 4.762500000000002842 ) ;
#88603=ORIENTED_EDGE ( 'NONE', *, *, #55345, .F. ) ;
#88605=EDGE_CURVE ( 'NONE', #45431, #32749, #6985, .T. ) ;
#88622=DIRECTION ( 'NONE',  ( 1.000000000000000000, 0.000000000000000000, 0.000000000000000000 ) ) ;
#88630=VERTEX_POINT ( 'NONE', #85100 ) ;
#88679=CARTESIAN_POINT ( 'NONE',  ( -487.2989999999999782, 7.143750000000339995, 6.988054014476278830 ) ) ;
#88680=ADVANCED_FACE ( 'NONE', ( #609 ), #55544, .T. ) ;
#88751=CARTESIAN_POINT ( 'NONE',  ( -53.64297985755450782, 53.97500000000000142, 70.79999999999999716 ) ) ;
#88760=FILL_AREA_STYLE_COLOUR ( '', #8595 ) ;
#88796=CARTESIAN_POINT ( 'NONE',  ( -48.02966122971774610, 65.60000000000000853, -43.00307561052233751 ) ) ;
#88804=AXIS2_PLACEMENT_3D ( 'NONE', #3031, #30731, #86153 ) ;
#88807=ORIENTED_EDGE ( 'NONE', *, *, #4086, .T. ) ;
#88810=CARTESIAN_POINT ( 'NONE',  ( 0.000000000000000000, 100.5999999999999659, 0.000000000000000000 ) ) ;
#88834=LINE ( 'NONE', #67924, #84499 ) ;
#88846=ADVANCED_FACE ( 'NONE', ( #17377 ), #36929, .F. ) ;
#88848=ORIENTED_EDGE ( 'NONE', *, *, #7852, .F. ) ;
#88864=ORIENTED_EDGE ( 'NONE', *, *, #84809, .T. ) ;
#88871=CARTESIAN_POINT ( 'NONE',  ( -254.0000000000000000, 3.174999999999999822, -41.27499999999999858 ) ) ;
#88877=ORIENTED_EDGE ( 'NONE', *, *, #58100, .T. ) ;
#88880=EDGE_CURVE ( 'NONE', #88630, #77919, #10555, .T. ) ;
#88907=DIRECTION ( 'NONE',  ( 0.000000000000000000, 0.000000000000000000, -1.000000000000000000 ) ) ;
#88923=FACE_OUTER_BOUND ( 'NONE', #49225, .T. ) ;
#88925=ADVANCED_FACE ( 'NONE', ( #36335, #57205 ), #78586, .T. ) ;
#88944=DIRECTION ( 'NONE',  ( -0.9770521142508956647, -1.387778780781445676E-17, 0.2130003897598659324 ) ) ;
#88961=DIRECTION ( 'NONE',  ( -1.000000000000000000, 0.000000000000000000, 0.000000000000000000 ) ) ;
#88996=ADVANCED_BREP_SHAPE_REPRESENTATION ( '', ( #47652, #50656 ), #27649 ) ;
#89008=CIRCLE ( 'NONE', #20858, 17.33514202138210791 ) ;
#89024=VECTOR ( 'NONE', #66169, 999.9999999999998863 ) ;
#89030=B_SPLINE_CURVE_WITH_KNOTS ( 'NONE', 1,
 ( #45994, #73726 ),
 .UNSPECIFIED., .F., .F.,
 ( 2, 2 ),
 ( 0.000000000000000000, 0.002370257936674861985 ),
 .UNSPECIFIED. ) ;
#89060=CARTESIAN_POINT ( 'NONE',  ( 0.000000000000000000, 65.60000000000000853, 0.000000000000000000 ) ) ;
#89081=CARTESIAN_POINT ( 'NONE',  ( -446.0240000000000009, 53.97500000000000142, 50.79999999999999716 ) ) ;
#89104=CARTESIAN_POINT ( 'NONE',  ( -1.651467058941123778, 70.03175547422245018, 118.3472173295736951 ) ) ;
#89107=FACE_OUTER_BOUND ( 'NONE', #58901, .T. ) ;
#89167=CARTESIAN_POINT ( 'NONE',  ( -487.2989999999999782, 7.143750000000339995, 6.988054014476278830 ) ) ;
#89219=EDGE_CURVE ( 'NONE', #63134, #1004, #79361, .T. ) ;
#89243=CARTESIAN_POINT ( 'NONE',  ( -47.18030668273772221, 93.07500000000001705, 75.34738655934135920 ) ) ;
#89251=EDGE_CURVE ( 'NONE', #63134, #9022, #12988, .T. ) ;
#89269=DIRECTION ( 'NONE',  ( -0.000000000000000000, 0.8660254037844382635, 0.5000000000000008882 ) ) ;
#89273=VECTOR ( 'NONE', #47852, 1000.000000000000114 ) ;
#89278=ORIENTED_EDGE ( 'NONE', *, *, #26702, .T. ) ;
#89304=DIRECTION ( 'NONE',  ( 0.000000000000000000, 0.000000000000000000, 1.000000000000000000 ) ) ;
#89347=AXIS2_PLACEMENT_3D ( 'NONE', #13691, #69559, #20523 ) ;
#89349=ORIENTED_EDGE ( 'NONE', *, *, #28041, .F. ) ;
#89365=CARTESIAN_POINT ( 'NONE',  ( -41.60202597009397607, 65.59999999999998010, 50.85338361873603219 ) ) ;
#89367=DIRECTION ( 'NONE',  ( 1.000000000000000000, 0.000000000000000000, 0.000000000000000000 ) ) ;
#89385=ORIENTED_EDGE ( 'NONE', *, *, #33785, .T. ) ;
#89401=VECTOR ( 'NONE', #87443, 1000.000000000000000 ) ;
#89421=CARTESIAN_POINT ( 'NONE',  ( 68.86456684384336313, 93.07500000000001705, 56.22171674193015889 ) ) ;
#89454=DIRECTION ( 'NONE',  ( -1.000000000000000000, 0.000000000000000000, 0.000000000000000000 ) ) ;
#89481=DIRECTION ( 'NONE',  ( 2.081668171172168119E-15, 0.000000000000000000, -1.000000000000000000 ) ) ;
#89496=DIRECTION ( 'NONE',  ( 0.000000000000000000, 0.7071067811865378028, 0.7071067811865573427 ) ) ;
#89514=DIRECTION ( 'NONE',  ( 0.000000000000000000, 1.000000000000000000, 0.000000000000000000 ) ) ;
#89520=DIRECTION ( 'NONE',  ( -1.000000000000000000, 0.000000000000000000, 0.000000000000000000 ) ) ;
#89543=ORIENTED_EDGE ( 'NONE', *, *, #48192, .F. ) ;
#89566=AXIS2_PLACEMENT_3D ( 'NONE', #629, #34255, #84671 ) ;
#89582=DIRECTION ( 'NONE',  ( 0.000000000000000000, 0.000000000000000000, -1.000000000000000000 ) ) ;
#89620=CARTESIAN_POINT ( 'NONE',  ( 0.000000000000000000, 91.07499999999996021, 0.000000000000000000 ) ) ;
#89641=DIRECTION ( 'NONE',  ( -0.8660254037844420383, -0.4999999999999941158, 0.000000000000000000 ) ) ;
#89643=FACE_OUTER_BOUND ( 'NONE', #79887, .T. ) ;
#89656=CARTESIAN_POINT ( 'NONE',  ( 0.000000000000000000, 0.000000000000000000, 0.000000000000000000 ) ) ;
#89688=ADVANCED_FACE ( 'NONE', ( #77145 ), #66744, .T. ) ;
#89689=LINE ( 'NONE', #76944, #47151 ) ;
#89746=ORIENTED_EDGE ( 'NONE', *, *, #12450, .F. ) ;
#89801=ORIENTED_EDGE ( 'NONE', *, *, #31824, .T. ) ;
#89825=CARTESIAN_POINT ( 'NONE',  ( -492.0614999999999668, 14.28750000000026077, 15.87499999999969802 ) ) ;
#89831=VECTOR ( 'NONE', #71460, 1000.000000000000000 ) ;
#89833=CARTESIAN_POINT ( 'NONE',  ( -53.92625078532105931, 53.97500000000000142, 70.79999999999999716 ) ) ;
#89859=ORIENTED_EDGE ( 'NONE', *, *, #48623, .F. ) ;
#89873=DIRECTION ( 'NONE',  ( 0.000000000000000000, 0.000000000000000000, -1.000000000000000000 ) ) ;
#89902=ORIENTED_EDGE ( 'NONE', *, *, #56428, .T. ) ;
#89904=EDGE_LOOP ( 'NONE', ( #31411, #79118 ) ) ;
#89921=ORIENTED_EDGE ( 'NONE', *, *, #9959, .T. ) ;
ENDSEC;
END-ISO-10303-21;
